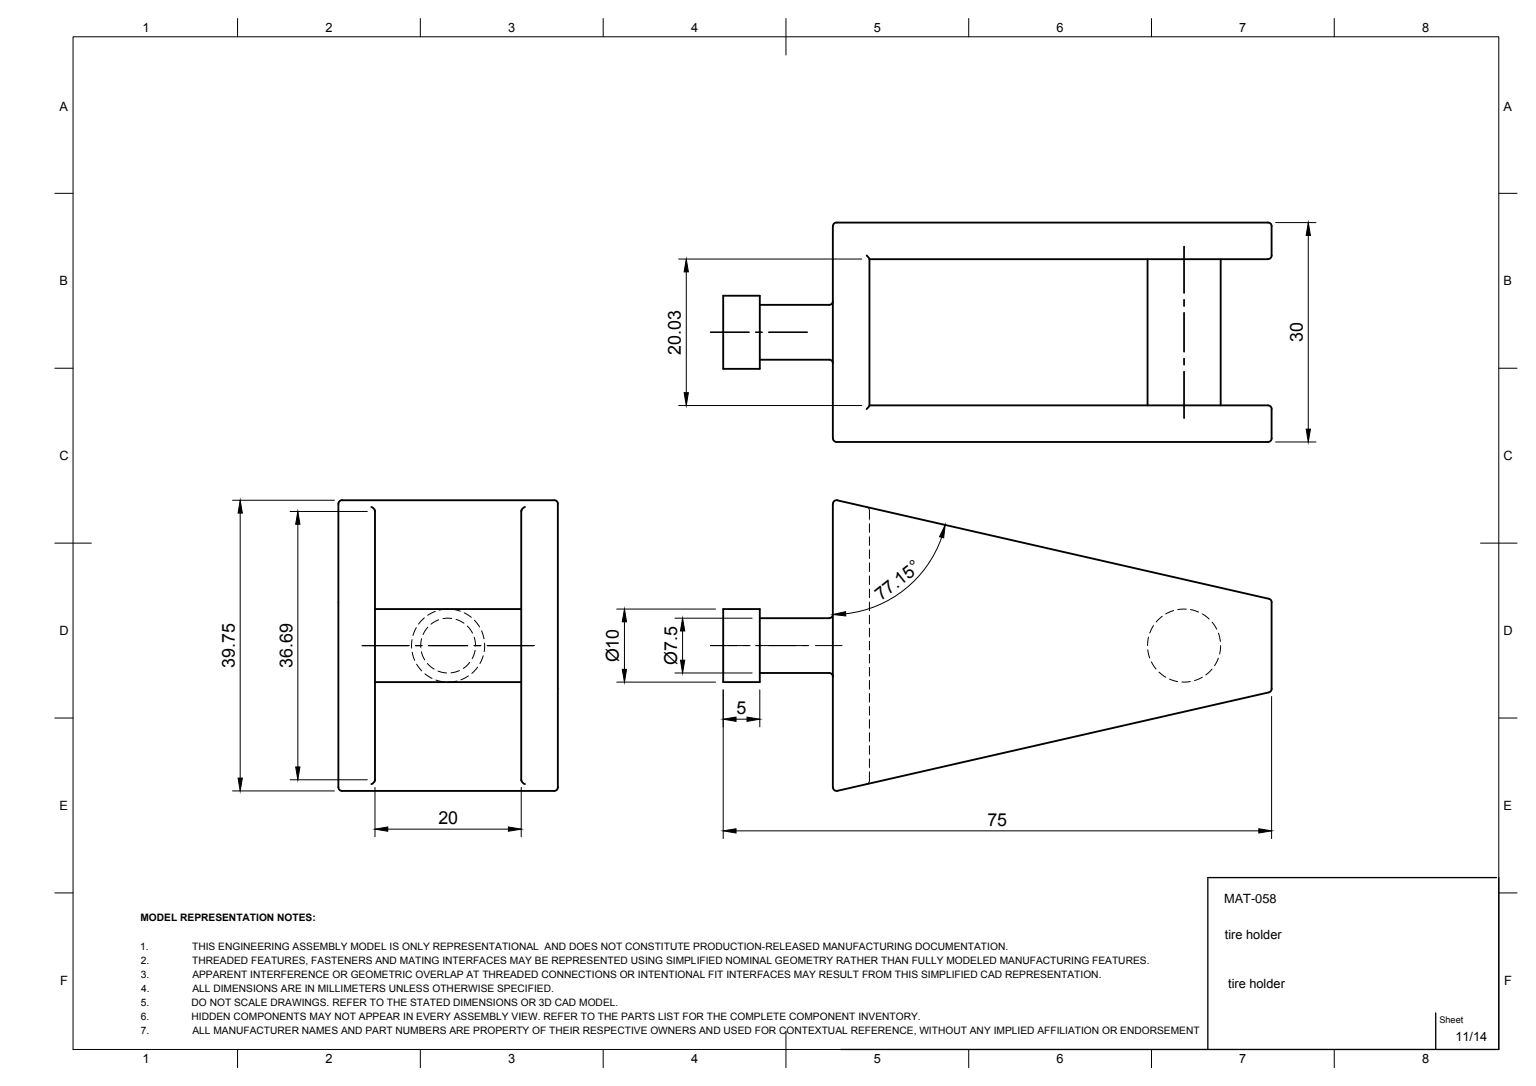
ISO-10303-21;
HEADER;
FILE_DESCRIPTION (('STEP AP214'),
    '1' );
FILE_NAME ('tire holder.step',
    '2026-10-21T17:54:40',
    ( '' ),
    ( '' ),
    'SwSTEP 2.0',
    'SolidWorks 2026',
    '' );
FILE_SCHEMA (( 'AUTOMOTIVE_DESIGN' ));
ENDSEC;

DATA;
#45=LINE ( 'NONE', #24156, #46879 ) ;
#75=DIRECTION ( 'NONE',  ( 0.000000000000000000, 3.469446951953611033E-15, 1.000000000000000000 ) ) ;
#80=CARTESIAN_POINT ( 'NONE',  ( -10.00000000000000355, -34.54492135858216528, 5.000000000000000000 ) ) ;
#120=EDGE_LOOP ( 'NONE', ( #42684, #24578, #28599, #31905 ) ) ;
#171=EDGE_LOOP ( 'NONE', ( #28708, #6316, #9774, #15681 ) ) ;
#207=DIRECTION ( 'NONE',  ( -3.469446951953610639E-15, 0.000000000000000000, 1.000000000000000000 ) ) ;
#240=AXIS2_PLACEMENT_3D ( 'NONE', #22049, #38489, #34625 ) ;
#261=LINE ( 'NONE', #24365, #22339 ) ;
#263=FACE_OUTER_BOUND ( 'NONE', #4989, .T. ) ;
#284=AXIS2_PLACEMENT_3D ( 'NONE', #31805, #27184, #19732 ) ;
#316=AXIS2_PLACEMENT_3D ( 'NONE', #35851, #27117, #42740 ) ;
#348=DIRECTION ( 'NONE',  ( -1.000000000000000000, -0.000000000000000000, -0.000000000000000000 ) ) ;
#396=AXIS2_PLACEMENT_3D ( 'NONE', #30919, #46501, #11395 ) ;
#430=LINE ( 'NONE', #46568, #36748 ) ;
#460=ORIENTED_EDGE ( 'NONE', *, *, #7056, .F. ) ;
#535=FACE_OUTER_BOUND ( 'NONE', #48692, .T. ) ;
#576=VERTEX_POINT ( 'NONE', #29130 ) ;
#579=DIRECTION ( 'NONE',  ( -1.000000000000000000, 0.000000000000000000, 0.000000000000000000 ) ) ;
#589=CARTESIAN_POINT ( 'NONE',  ( -10.49999999999999467, -46.01315789473684248, -5.916985404131818171 ) ) ;
#592=EDGE_CURVE ( 'NONE', #28510, #10704, #32994, .T. ) ;
#599=DIRECTION ( 'NONE',  ( 0.000000000000000000, 0.2223603367690637489, -0.9749645535258953943 ) ) ;
#609=VERTEX_POINT ( 'NONE', #32230 ) ;
#633=FACE_OUTER_BOUND ( 'NONE', #3064, .T. ) ;
#751=FACE_OUTER_BOUND ( 'NONE', #17565, .T. ) ;
#819=EDGE_LOOP ( 'NONE', ( #45356, #48998, #15248, #7254 ) ) ;
#834=LINE ( 'NONE', #43911, #33679 ) ;
#877=CARTESIAN_POINT ( 'NONE',  ( 9.999999999999998224, -41.51315789473684248, -25.00000000000000000 ) ) ;
#894=LINE ( 'NONE', #40643, #19792 ) ;
#895=ORIENTED_EDGE ( 'NONE', *, *, #4687, .F. ) ;
#954=CARTESIAN_POINT ( 'NONE',  ( 10.00419011302946259, 8.486842105263161073, 18.42339408367722697 ) ) ;
#973=CARTESIAN_POINT ( 'NONE',  ( -10.01251772323708522, 8.486842105263161073, -18.46084505325461578 ) ) ;
#990=CARTESIAN_POINT ( 'NONE',  ( 15.00000000000000000, 8.986842105263161073, 18.46084505325461578 ) ) ;
#1024=DIRECTION ( 'NONE',  ( 0.000000000000000000, 0.000000000000000000, -1.000000000000000000 ) ) ;
#1096=DIRECTION ( 'NONE',  ( 1.000000000000000000, -0.000000000000000000, -0.000000000000000000 ) ) ;
#1116=EDGE_CURVE ( 'NONE', #10525, #16010, #26971, .T. ) ;
#1161=VERTEX_POINT ( 'NONE', #21613 ) ;
#1182=SPHERICAL_SURFACE ( 'NONE', #12671, 0.5000000000000000000 ) ;
#1197=DIRECTION ( 'NONE',  ( 0.000000000000000000, -0.000000000000000000, 1.000000000000000000 ) ) ;
#1232=CARTESIAN_POINT ( 'NONE',  ( 14.49999999999999822, 12.98684210526315930, 19.37312575500899925 ) ) ;
#1234=DIRECTION ( 'NONE',  ( -0.000000000000000000, -1.000000000000000000, -0.000000000000000000 ) ) ;
#1240=EDGE_CURVE ( 'NONE', #38020, #13837, #23637, .T. ) ;
#1272=ORIENTED_EDGE ( 'NONE', *, *, #4241, .T. ) ;
#1288=ORIENTED_EDGE ( 'NONE', *, *, #47195, .F. ) ;
#1496=DIRECTION ( 'NONE',  ( 0.000000000000000000, 0.000000000000000000, -1.000000000000000000 ) ) ;
#1555=ORIENTED_EDGE ( 'NONE', *, *, #40015, .F. ) ;
#1561=ADVANCED_FACE ( 'NONE', ( #6652 ), #17704, .T. ) ;
#1634=VECTOR ( 'NONE', #50677, 1000.000000000000000 ) ;
#1646=CIRCLE ( 'NONE', #12289, 0.4999999999999997224 ) ;
#1662=VERTEX_POINT ( 'NONE', #15882 ) ;
#1709=DIRECTION ( 'NONE',  ( 0.000000000000000000, 6.938893903907221278E-15, -1.000000000000000000 ) ) ;
#1723=DIRECTION ( 'NONE',  ( -1.542934785277626909E-15, 0.9749645535258950613, 0.2223603367690656918 ) ) ;
#1780=AXIS2_PLACEMENT_3D ( 'NONE', #25486, #49289, #14172 ) ;
#1792=EDGE_CURVE ( 'NONE', #35881, #24944, #10954, .T. ) ;
#1843=CIRCLE ( 'NONE', #32181, 0.4999999999999997224 ) ;
#1845=ORIENTED_EDGE ( 'NONE', *, *, #9182, .T. ) ;
#1941=DIRECTION ( 'NONE',  ( 0.000000000000000000, 0.000000000000000000, -1.000000000000000000 ) ) ;
#2025=CARTESIAN_POINT ( 'NONE',  ( 4.592425496802573972E-16, 23.48684210526316107, 3.750000000000000000 ) ) ;
#2046=EDGE_LOOP ( 'NONE', ( #43481, #9210, #37838, #21818, #19453, #27829, #8404, #30225 ) ) ;
#2075=ADVANCED_FACE ( 'NONE', ( #43515 ), #35854, .T. ) ;
#2076=ORIENTED_EDGE ( 'NONE', *, *, #10770, .F. ) ;
#2264=CARTESIAN_POINT ( 'NONE',  ( -10.01251772323708700, 8.486842105263161073, 18.46084505325461578 ) ) ;
#2383=CYLINDRICAL_SURFACE ( 'NONE', #27076, 0.5000000000000004441 ) ;
#2455=AXIS2_PLACEMENT_3D ( 'NONE', #15350, #35622, #7647 ) ;
#2478=ORIENTED_EDGE ( 'NONE', *, *, #4027, .F. ) ;
#2494=( BOUNDED_CURVE ( )  B_SPLINE_CURVE ( 3, ( #33761, #6547, #22202, #15008 ),
 .UNSPECIFIED., .F., .F. ) 
 B_SPLINE_CURVE_WITH_KNOTS ( ( 4, 4 ),
 ( 1.346561575685802925, 1.570796326794893671 ),
 .UNSPECIFIED. ) 
 CURVE ( )  GEOMETRIC_REPRESENTATION_ITEM ( )  RATIONAL_B_SPLINE_CURVE ( ( 1.000000000000000000, 0.9958142854328209115, 0.9958142854328209115, 1.000000000000000000 ) ) 
 REPRESENTATION_ITEM ( '' )  );
#2510=ORIENTED_EDGE ( 'NONE', *, *, #26162, .F. ) ;
#2540=AXIS2_PLACEMENT_3D ( 'NONE', #23259, #35857, #19920 ) ;
#2581=DIRECTION ( 'NONE',  ( 1.000000000000000000, -0.000000000000000000, -0.000000000000000000 ) ) ;
#2605=ADVANCED_FACE ( 'NONE', ( #535 ), #28227, .T. ) ;
#2654=VECTOR ( 'NONE', #49924, 1000.000000000000000 ) ;
#2662=ORIENTED_EDGE ( 'NONE', *, *, #17111, .T. ) ;
#2697=CARTESIAN_POINT ( 'NONE',  ( -9.999999999999994671, -46.01315789473684248, -5.916985404131814619 ) ) ;
#2752=DIRECTION ( 'NONE',  ( 0.000000000000000000, 0.000000000000000000, 1.000000000000000000 ) ) ;
#2761=EDGE_CURVE ( 'NONE', #42454, #20304, #29988, .T. ) ;
#2842=CARTESIAN_POINT ( 'NONE',  ( -15.00000000000000000, 12.98684210526315930, -20.00000000000000000 ) ) ;
#2857=LINE ( 'NONE', #42115, #24978 ) ;
#2930=AXIS2_PLACEMENT_3D ( 'NONE', #5505, #48309, #9612 ) ;
#2932=FACE_OUTER_BOUND ( 'NONE', #31942, .T. ) ;
#2933=( BOUNDED_CURVE ( )  B_SPLINE_CURVE ( 3, ( #26666, #25209, #13891, #30775 ),
 .UNSPECIFIED., .F., .F. ) 
 B_SPLINE_CURVE_WITH_KNOTS ( ( 4, 4 ),
 ( 1.570796326794886788, 1.795031077903984418 ),
 .UNSPECIFIED. ) 
 CURVE ( )  GEOMETRIC_REPRESENTATION_ITEM ( )  RATIONAL_B_SPLINE_CURVE ( ( 1.000000000000000000, 0.9958142854328206894, 0.9958142854328206894, 1.000000000000000000 ) ) 
 REPRESENTATION_ITEM ( '' )  );
#2949=SPHERICAL_SURFACE ( 'NONE', #43069, 0.5000000000000000000 ) ;
#2968=EDGE_LOOP ( 'NONE', ( #14933, #7197, #19117, #5943 ) ) ;
#3064=EDGE_LOOP ( 'NONE', ( #38905, #19899, #45220, #15309 ) ) ;
#3066=VERTEX_POINT ( 'NONE', #25504 ) ;
#3104=ORIENTED_EDGE ( 'NONE', *, *, #47830, .T. ) ;
#3173=CYLINDRICAL_SURFACE ( 'NONE', #24749, 0.5000000000000007772 ) ;
#3180=CARTESIAN_POINT ( 'NONE',  ( -14.49999999999999822, 12.98684210526315930, -19.37312575500900280 ) ) ;
#3200=CARTESIAN_POINT ( 'NONE',  ( -10.01251772323708700, 8.486842105263161073, 18.46084505325461578 ) ) ;
#3209=DIRECTION ( 'NONE',  ( 0.000000000000000000, 0.000000000000000000, -1.000000000000000000 ) ) ;
#3241=EDGE_CURVE ( 'NONE', #43437, #39173, #48510, .T. ) ;
#3301=CIRCLE ( 'NONE', #17237, 5.000000000000000000 ) ;
#3396=EDGE_CURVE ( 'NONE', #19221, #42182, #41183, .T. ) ;
#3427=( NAMED_UNIT ( * ) PLANE_ANGLE_UNIT ( ) SI_UNIT ( $, .RADIAN. ) );
#3464=CIRCLE ( 'NONE', #8400, 0.4999999999999995559 ) ;
#3536=EDGE_CURVE ( 'NONE', #24944, #35881, #21519, .T. ) ;
#3663=ORIENTED_EDGE ( 'NONE', *, *, #7740, .F. ) ;
#3712=ORIENTED_EDGE ( 'NONE', *, *, #33824, .F. ) ;
#3728=DIRECTION ( 'NONE',  ( 0.000000000000000000, 0.000000000000000000, 1.000000000000000000 ) ) ;
#3770=CARTESIAN_POINT ( 'NONE',  ( -14.49999999999999822, 13.59802227364769323, -19.51251772323705325 ) ) ;
#3785=ORIENTED_EDGE ( 'NONE', *, *, #26162, .T. ) ;
#3786=EDGE_LOOP ( 'NONE', ( #5766, #9145, #25506, #27864 ) ) ;
#3830=CARTESIAN_POINT ( 'NONE',  ( 10.00000000000000355, -48.43825625180578953, 5.363892796379245986 ) ) ;
#3840=DIRECTION ( 'NONE',  ( -1.000000000000000000, -0.000000000000000000, -0.000000000000000000 ) ) ;
#3855=EDGE_CURVE ( 'NONE', #35640, #27759, #5651, .T. ) ;
#3910=UNCERTAINTY_MEASURE_WITH_UNIT (LENGTH_MEASURE( 1.000000000000000082E-05 ), #38612, 'distance_accuracy_value', 'NONE');
#3932=ORIENTED_EDGE ( 'NONE', *, *, #33759, .F. ) ;
#3990=CARTESIAN_POINT ( 'NONE',  ( 15.00000000000000000, -46.01315789473684248, 0.000000000000000000 ) ) ;
#4021=VECTOR ( 'NONE', #29786, 1000.000000000000000 ) ;
#4027=EDGE_CURVE ( 'NONE', #23110, #34075, #10732, .T. ) ;
#4062=ORIENTED_EDGE ( 'NONE', *, *, #44355, .T. ) ;
#4075=FACE_OUTER_BOUND ( 'NONE', #46172, .T. ) ;
#4085=DIRECTION ( 'NONE',  ( -0.000000000000000000, 1.000000000000000000, 0.000000000000000000 ) ) ;
#4104=FACE_OUTER_BOUND ( 'NONE', #4399, .T. ) ;
#4145=FACE_OUTER_BOUND ( 'NONE', #18052, .T. ) ;
#4234=CYLINDRICAL_SURFACE ( 'NONE', #14707, 0.5000000000000004441 ) ;
#4241=EDGE_CURVE ( 'NONE', #24669, #43437, #22901, .T. ) ;
#4256=ORIENTED_EDGE ( 'NONE', *, *, #50333, .T. ) ;
#4260=AXIS2_PLACEMENT_3D ( 'NONE', #32923, #33666, #24959 ) ;
#4282=CARTESIAN_POINT ( 'NONE',  ( 10.25676241992214877, 8.638513918217338272, 18.89424093979656405 ) ) ;
#4395=DIRECTION ( 'NONE',  ( 0.000000000000000000, -0.2223603367690619725, -0.9749645535258958384 ) ) ;
#4399=EDGE_LOOP ( 'NONE', ( #26499, #28171, #23925, #10924 ) ) ;
#4431=CARTESIAN_POINT ( 'NONE',  ( 15.00000000000000000, 13.48684210526315930, 19.37312575500900280 ) ) ;
#4458=CIRCLE ( 'NONE', #13457, 0.5000000000000004441 ) ;
#4485=VECTOR ( 'NONE', #38359, 1000.000000000000000 ) ;
#4487=ORIENTED_EDGE ( 'NONE', *, *, #20206, .F. ) ;
#4544=LINE ( 'NONE', #24549, #10987 ) ;
#4626=AXIS2_PLACEMENT_3D ( 'NONE', #26012, #29596, #18790 ) ;
#4650=DIRECTION ( 'NONE',  ( 0.000000000000000000, 0.000000000000000000, 1.000000000000000000 ) ) ;
#4687=EDGE_CURVE ( 'NONE', #35926, #43437, #34948, .T. ) ;
#4718=DIRECTION ( 'NONE',  ( 1.000000000000000000, 6.938893903907233308E-16, 0.000000000000000000 ) ) ;
#4758=ORIENTED_EDGE ( 'NONE', *, *, #4027, .T. ) ;
#4779=CARTESIAN_POINT ( 'NONE',  ( 9.999999999999962697, 8.486842105263161073, 18.38522261288946780 ) ) ;
#4828=AXIS2_PLACEMENT_3D ( 'NONE', #3770, #19420, #15572 ) ;
#4835=VECTOR ( 'NONE', #39057, 1000.000000000000000 ) ;
#4900=DIRECTION ( 'NONE',  ( -6.938893903907221278E-15, -0.000000000000000000, -1.000000000000000000 ) ) ;
#4964=DIRECTION ( 'NONE',  ( 0.000000000000000000, -1.000000000000000000, 0.000000000000000000 ) ) ;
#4989=EDGE_LOOP ( 'NONE', ( #24819, #3104, #38758 ) ) ;
#4996=ORIENTED_EDGE ( 'NONE', *, *, #34082, .F. ) ;
#5053=LINE ( 'NONE', #17118, #10391 ) ;
#5074=DIRECTION ( 'NONE',  ( 1.000000000000000000, 0.000000000000000000, -0.000000000000000000 ) ) ;
#5167=AXIS2_PLACEMENT_3D ( 'NONE', #17587, #21943, #1941 ) ;
#5214=( LENGTH_UNIT ( ) NAMED_UNIT ( * ) SI_UNIT ( .MILLI., .METRE. ) );
#5228=DIRECTION ( 'NONE',  ( 0.000000000000000000, -0.9749645535258959494, -0.2223603367690620558 ) ) ;
#5249=ORIENTED_EDGE ( 'NONE', *, *, #39960, .F. ) ;
#5287=AXIS2_PLACEMENT_3D ( 'NONE', #877, #4718, #17016 ) ;
#5349=DIRECTION ( 'NONE',  ( -0.000000000000000000, 1.000000000000000000, 0.000000000000000000 ) ) ;
#5426=VERTEX_POINT ( 'NONE', #29943 ) ;
#5505=CARTESIAN_POINT ( 'NONE',  ( -14.49999999999999822, 12.98684210526315930, 19.37312575500900280 ) ) ;
#5556=VERTEX_POINT ( 'NONE', #32723 ) ;
#5562=DIRECTION ( 'NONE',  ( 0.000000000000000000, -0.2223603367690656640, 0.9749645535258950613 ) ) ;
#5568=EDGE_LOOP ( 'NONE', ( #49170, #12060, #17176 ) ) ;
#5569=DIRECTION ( 'NONE',  ( 0.000000000000000000, 1.000000000000000000, 0.000000000000000000 ) ) ;
#5605=DIRECTION ( 'NONE',  ( -0.000000000000000000, -1.000000000000000000, -0.000000000000000000 ) ) ;
#5606=EDGE_CURVE ( 'NONE', #32346, #49488, #6014, .T. ) ;
#5651=CIRCLE ( 'NONE', #37653, 0.4999999999999997224 ) ;
#5654=DIRECTION ( 'NONE',  ( -1.000000000000000000, 0.000000000000000000, 0.000000000000000000 ) ) ;
#5662=CARTESIAN_POINT ( 'NONE',  ( -14.49999999999999822, -46.01315789473684248, -5.916985404131818171 ) ) ;
#5718=AXIS2_PLACEMENT_3D ( 'NONE', #46898, #5349, #28463 ) ;
#5766=ORIENTED_EDGE ( 'NONE', *, *, #17761, .T. ) ;
#5824=VERTEX_POINT ( 'NONE', #13102 ) ;
#5861=ORIENTED_EDGE ( 'NONE', *, *, #25959, .F. ) ;
#5908=DIRECTION ( 'NONE',  ( -0.000000000000000000, 0.9749645535258953943, 0.2223603367690637489 ) ) ;
#5936=CARTESIAN_POINT ( 'NONE',  ( 10.50000000000000178, -46.12433806312137108, 6.404467680894761372 ) ) ;
#5940=CARTESIAN_POINT ( 'NONE',  ( 10.25676241992214344, 8.638513918217336496, -18.89424093979656760 ) ) ;
#5943=ORIENTED_EDGE ( 'NONE', *, *, #592, .F. ) ;
#6014=LINE ( 'NONE', #24519, #32174 ) ;
#6166=DIRECTION ( 'NONE',  ( -1.000000000000000000, 0.000000000000000000, -0.000000000000000000 ) ) ;
#6187=ORIENTED_EDGE ( 'NONE', *, *, #28725, .T. ) ;
#6196=PRODUCT_DEFINITION_FORMATION_WITH_SPECIFIED_SOURCE ( 'ANY', '', #26565, .NOT_KNOWN. ) ;
#6204=DIRECTION ( 'NONE',  ( 0.000000000000000000, 0.000000000000000000, 1.000000000000000000 ) ) ;
#6271=CARTESIAN_POINT ( 'NONE',  ( 15.00000000000000000, -46.01315789473684248, 5.916985404131816395 ) ) ;
#6278=CIRCLE ( 'NONE', #19373, 0.4999999999999995559 ) ;
#6285=CARTESIAN_POINT ( 'NONE',  ( -10.06660411345808193, 8.486842105263161073, -18.70408263333243326 ) ) ;
#6306=DIRECTION ( 'NONE',  ( -0.000000000000000000, 1.000000000000000000, 0.000000000000000000 ) ) ;
#6316=ORIENTED_EDGE ( 'NONE', *, *, #12510, .F. ) ;
#6317=FACE_OUTER_BOUND ( 'NONE', #44802, .T. ) ;
#6351=ORIENTED_EDGE ( 'NONE', *, *, #3536, .T. ) ;
#6366=CARTESIAN_POINT ( 'NONE',  ( -10.00000000000003375, 8.486842105263161073, 18.38522261288946780 ) ) ;
#6426=ADVANCED_FACE ( 'NONE', ( #7629 ), #43272, .T. ) ;
#6443=VERTEX_POINT ( 'NONE', #46577 ) ;
#6516=CARTESIAN_POINT ( 'NONE',  ( -14.49999999999999822, 12.87566193687862715, -19.86060803177194956 ) ) ;
#6530=AXIS2_PLACEMENT_3D ( 'NONE', #50614, #15762, #11667 ) ;
#6547=CARTESIAN_POINT ( 'NONE',  ( 10.00419011302945904, 8.486842105263161073, -18.42339408367723053 ) ) ;
#6652=FACE_OUTER_BOUND ( 'NONE', #35530, .T. ) ;
#6701=DIRECTION ( 'NONE',  ( 0.000000000000000000, 0.000000000000000000, -1.000000000000000000 ) ) ;
#6724=EDGE_LOOP ( 'NONE', ( #17001, #30815, #36441 ) ) ;
#6731=ORIENTED_EDGE ( 'NONE', *, *, #11598, .F. ) ;
#6774=CARTESIAN_POINT ( 'NONE',  ( 10.50000000000000178, -46.01315789473684248, -5.916985404131818171 ) ) ;
#6799=CARTESIAN_POINT ( 'NONE',  ( 0.000000000000000000, 23.48684210526316107, 0.000000000000000000 ) ) ;
#6871=DIRECTION ( 'NONE',  ( 0.000000000000000000, -1.000000000000000000, 0.000000000000000000 ) ) ;
#6885=CARTESIAN_POINT ( 'NONE',  ( 9.999999999999998224, 8.486842105263161073, 18.46084505325461933 ) ) ;
#6895=CARTESIAN_POINT ( 'NONE',  ( 9.999999999999998224, 8.486842105263161073, -18.46084505325461578 ) ) ;
#6946=DIRECTION ( 'NONE',  ( 6.938893903907233308E-16, -1.000000000000000000, 0.000000000000000000 ) ) ;
#6954=AXIS2_PLACEMENT_3D ( 'NONE', #9415, #12996, #49122 ) ;
#6956=ORIENTED_EDGE ( 'NONE', *, *, #7114, .F. ) ;
#6977=AXIS2_PLACEMENT_3D ( 'NONE', #21956, #45271, #37879 ) ;
#6998=AXIS2_PLACEMENT_3D ( 'NONE', #21667, #49075, #29623 ) ;
#7040=VECTOR ( 'NONE', #15019, 1000.000000000000000 ) ;
#7052=CARTESIAN_POINT ( 'NONE',  ( 4.592425496802573972E-16, 13.98684210526316107, 3.750000000000000000 ) ) ;
#7056=EDGE_CURVE ( 'NONE', #38020, #1662, #894, .T. ) ;
#7062=EDGE_CURVE ( 'NONE', #35881, #31952, #32188, .T. ) ;
#7084=ORIENTED_EDGE ( 'NONE', *, *, #10641, .F. ) ;
#7113=EDGE_CURVE ( 'NONE', #7866, #1662, #37840, .T. ) ;
#7114=EDGE_CURVE ( 'NONE', #20701, #39523, #30456, .T. ) ;
#7197=ORIENTED_EDGE ( 'NONE', *, *, #25233, .F. ) ;
#7202=DIRECTION ( 'NONE',  ( -1.000000000000000000, -6.938893903907233308E-16, 0.000000000000000000 ) ) ;
#7254=ORIENTED_EDGE ( 'NONE', *, *, #24579, .F. ) ;
#7273=EDGE_CURVE ( 'NONE', #28229, #5824, #15967, .T. ) ;
#7275=FACE_OUTER_BOUND ( 'NONE', #21467, .T. ) ;
#7324=ORIENTED_EDGE ( 'NONE', *, *, #31534, .F. ) ;
#7325=EDGE_LOOP ( 'NONE', ( #22359, #3712, #17058, #14186 ) ) ;
#7392=EDGE_LOOP ( 'NONE', ( #23020, #17478, #31410, #21280 ) ) ;
#7412=ORIENTED_EDGE ( 'NONE', *, *, #24326, .T. ) ;
#7417=EDGE_CURVE ( 'NONE', #16010, #39173, #12121, .T. ) ;
#7478=EDGE_CURVE ( 'NONE', #39523, #20701, #16513, .T. ) ;
#7479=CARTESIAN_POINT ( 'NONE',  ( 15.00000000000000000, -46.12433806312137108, -6.404467680894764925 ) ) ;
#7526=CARTESIAN_POINT ( 'NONE',  ( 15.00000000000000000, -3.557843729863134463, -15.59977635401528850 ) ) ;
#7618=AXIS2_PLACEMENT_3D ( 'NONE', #12378, #348, #43665 ) ;
#7629=FACE_OUTER_BOUND ( 'NONE', #7392, .T. ) ;
#7647=DIRECTION ( 'NONE',  ( 0.000000000000000000, 0.2223603367690619725, -0.9749645535258958384 ) ) ;
#7664=EDGE_CURVE ( 'NONE', #34755, #31952, #12256, .T. ) ;
#7676=DIRECTION ( 'NONE',  ( 1.000000000000000000, 0.000000000000000000, -1.734723475976805517E-15 ) ) ;
#7703=AXIS2_PLACEMENT_3D ( 'NONE', #8195, #4085, #8448 ) ;
#7731=ORIENTED_EDGE ( 'NONE', *, *, #23304, .T. ) ;
#7733=DIRECTION ( 'NONE',  ( -0.000000000000000000, 0.000000000000000000, -1.000000000000000000 ) ) ;
#7740=EDGE_CURVE ( 'NONE', #13837, #42454, #28716, .T. ) ;
#7746=DIRECTION ( 'NONE',  ( 1.542934785277601468E-15, 0.9749645535258959494, -0.2223603367690620558 ) ) ;
#7780=CIRCLE ( 'NONE', #36463, 0.5000000000000000000 ) ;
#7798=DIRECTION ( 'NONE',  ( 6.765175596986472868E-16, -0.9749645535258953943, -0.2223603367690637489 ) ) ;
#7806=LINE ( 'NONE', #43436, #23351 ) ;
#7809=ORIENTED_EDGE ( 'NONE', *, *, #25233, .T. ) ;
#7813=DIRECTION ( 'NONE',  ( 0.000000000000000000, 0.000000000000000000, 1.000000000000000000 ) ) ;
#7820=CARTESIAN_POINT ( 'NONE',  ( -14.49999999999999822, -46.51315789473684248, -5.916985404131818171 ) ) ;
#7828=LINE ( 'NONE', #35042, #44206 ) ;
#7829=ORIENTED_EDGE ( 'NONE', *, *, #36041, .T. ) ;
#7842=ORIENTED_EDGE ( 'NONE', *, *, #44186, .T. ) ;
#7866=VERTEX_POINT ( 'NONE', #30673 ) ;
#7886=AXIS2_PLACEMENT_3D ( 'NONE', #1232, #1723, #5562 ) ;
#7900=FACE_OUTER_BOUND ( 'NONE', #31199, .T. ) ;
#7910=VECTOR ( 'NONE', #1096, 1000.000000000000000 ) ;
#7922=ORIENTED_EDGE ( 'NONE', *, *, #13439, .T. ) ;
#8033=DIRECTION ( 'NONE',  ( 0.000000000000000000, 0.000000000000000000, 1.000000000000000000 ) ) ;
#8051=ADVANCED_FACE ( 'NONE', ( #47541 ), #4234, .T. ) ;
#8052=EDGE_CURVE ( 'NONE', #40121, #28181, #11932, .T. ) ;
#8082=EDGE_LOOP ( 'NONE', ( #35213, #15987, #29822, #26821, #47039, #4758, #23954, #45682 ) ) ;
#8195=CARTESIAN_POINT ( 'NONE',  ( 14.49999999999999822, -46.01315789473684248, 5.916985404131813731 ) ) ;
#8236=VERTEX_POINT ( 'NONE', #33954 ) ;
#8245=DIRECTION ( 'NONE',  ( -1.000000000000000000, 0.000000000000000000, 0.000000000000000000 ) ) ;
#8352=DIRECTION ( 'NONE',  ( 0.000000000000000000, 8.673617379884027583E-15, 1.000000000000000000 ) ) ;
#8358=ORIENTED_EDGE ( 'NONE', *, *, #46516, .F. ) ;
#8400=AXIS2_PLACEMENT_3D ( 'NONE', #50720, #35396, #28186 ) ;
#8402=EDGE_LOOP ( 'NONE', ( #48506, #22576, #41484 ) ) ;
#8404=ORIENTED_EDGE ( 'NONE', *, *, #23196, .T. ) ;
#8407=AXIS2_PLACEMENT_3D ( 'NONE', #16644, #35162, #43084 ) ;
#8416=EDGE_CURVE ( 'NONE', #12918, #28229, #15215, .T. ) ;
#8440=CARTESIAN_POINT ( 'NONE',  ( -10.49999999999999467, -46.01315789473684248, 5.916985404131814619 ) ) ;
#8448=DIRECTION ( 'NONE',  ( 3.469446951953616950E-15, 0.000000000000000000, -1.000000000000000000 ) ) ;
#8470=DIRECTION ( 'NONE',  ( 0.000000000000000000, 0.000000000000000000, 1.000000000000000000 ) ) ;
#8504=EDGE_CURVE ( 'NONE', #12400, #26840, #1646, .T. ) ;
#8514=CIRCLE ( 'NONE', #15903, 0.5000000000000004441 ) ;
#8582=DIRECTION ( 'NONE',  ( 6.765175596986471882E-16, -0.9749645535258953943, -0.2223603367690637489 ) ) ;
#8678=DIRECTION ( 'NONE',  ( 0.000000000000000000, 0.2223603367690656640, 0.9749645535258950613 ) ) ;
#8706=UNCERTAINTY_MEASURE_WITH_UNIT (LENGTH_MEASURE( 1.000000000000000082E-05 ), #5214, 'distance_accuracy_value', 'NONE');
#8869=ORIENTED_EDGE ( 'NONE', *, *, #24926, .F. ) ;
#8880=EDGE_CURVE ( 'NONE', #31952, #34755, #39343, .T. ) ;
#8920=DIRECTION ( 'NONE',  ( 0.000000000000000000, 0.000000000000000000, 1.000000000000000000 ) ) ;
#8941=CARTESIAN_POINT ( 'NONE',  ( 10.50000000000000178, -46.01315789473684248, -5.916985404131818171 ) ) ;
#8967=DIRECTION ( 'NONE',  ( 0.000000000000000000, 1.000000000000000000, -0.000000000000000000 ) ) ;
#8972=ADVANCED_FACE ( 'NONE', ( #18419 ), #25886, .T. ) ;
#9003=AXIS2_PLACEMENT_3D ( 'NONE', #31247, #43526, #30993 ) ;
#9016=ORIENTED_EDGE ( 'NONE', *, *, #11598, .T. ) ;
#9033=DIRECTION ( 'NONE',  ( -1.542934785277601468E-15, -0.9749645535258959494, 0.2223603367690620558 ) ) ;
#9040=CARTESIAN_POINT ( 'NONE',  ( 14.49999999999999822, 12.98684210526315930, -19.87312575500900280 ) ) ;
#9100=EDGE_CURVE ( 'NONE', #576, #5426, #31909, .T. ) ;
#9103=ORIENTED_EDGE ( 'NONE', *, *, #33702, .F. ) ;
#9111=ORIENTED_EDGE ( 'NONE', *, *, #23050, .T. ) ;
#9145=ORIENTED_EDGE ( 'NONE', *, *, #14539, .F. ) ;
#9163=DIRECTION ( 'NONE',  ( 1.000000000000000000, 0.000000000000000000, 0.000000000000000000 ) ) ;
#9182=EDGE_CURVE ( 'NONE', #5824, #26840, #26050, .T. ) ;
#9195=DIRECTION ( 'NONE',  ( -1.224646799147352468E-16, 0.000000000000000000, -1.000000000000000000 ) ) ;
#9210=ORIENTED_EDGE ( 'NONE', *, *, #25817, .T. ) ;
#9211=SPHERICAL_SURFACE ( 'NONE', #29493, 0.5000000000000000000 ) ;
#9268=CIRCLE ( 'NONE', #28932, 0.5000000000000004441 ) ;
#9298=PLANE ( 'NONE',  #30473 ) ;
#9406=ORIENTED_EDGE ( 'NONE', *, *, #29481, .T. ) ;
#9415=CARTESIAN_POINT ( 'NONE',  ( 15.00000000000000000, 12.98684210526315752, 19.37312575500900280 ) ) ;
#9419=DIRECTION ( 'NONE',  ( 0.000000000000000000, 0.000000000000000000, 1.000000000000000000 ) ) ;
#9431=CYLINDRICAL_SURFACE ( 'NONE', #38867, 0.5000000000000004441 ) ;
#9438=STYLED_ITEM('',(#50775),#22320);
#9462=DIRECTION ( 'NONE',  ( -1.000000000000000000, 0.000000000000000000, -0.000000000000000000 ) ) ;
#9479=VERTEX_POINT ( 'NONE', #20570 ) ;
#9512=DIRECTION ( 'NONE',  ( -1.000000000000000000, 0.000000000000000000, 6.938893903907222067E-15 ) ) ;
#9543=CARTESIAN_POINT ( 'NONE',  ( 15.00000000000000000, -46.01315789473684248, -5.916985404131813731 ) ) ;
#9570=EDGE_CURVE ( 'NONE', #19221, #30619, #25947, .T. ) ;
#9612=DIRECTION ( 'NONE',  ( 0.000000000000000000, 0.000000000000000000, 1.000000000000000000 ) ) ;
#9626=DIRECTION ( 'NONE',  ( 0.000000000000000000, 0.000000000000000000, 1.000000000000000000 ) ) ;
#9628=CARTESIAN_POINT ( 'NONE',  ( -15.00000000000000000, 13.59802227364770388, 19.51251772323705325 ) ) ;
#9651=DIRECTION ( 'NONE',  ( 1.000000000000000000, -0.000000000000000000, 0.000000000000000000 ) ) ;
#9717=CYLINDRICAL_SURFACE ( 'NONE', #12761, 5.000000000000000000 ) ;
#9731=PRODUCT_DEFINITION_SHAPE ( 'NONE', 'NONE',  #48451 ) ;
#9760=EDGE_LOOP ( 'NONE', ( #39795, #29788, #24517 ) ) ;
#9774=ORIENTED_EDGE ( 'NONE', *, *, #34082, .T. ) ;
#9854=CIRCLE ( 'NONE', #2455, 0.4999999999999997224 ) ;
#9855=EDGE_CURVE ( 'NONE', #20536, #16093, #25815, .T. ) ;
#9859=CIRCLE ( 'NONE', #38563, 0.4999999999999997224 ) ;
#9882=ADVANCED_FACE ( 'NONE', ( #6317 ), #2949, .T. ) ;
#9892=CIRCLE ( 'NONE', #26276, 0.5000000000000004441 ) ;
#9915=LINE ( 'NONE', #26074, #11981 ) ;
#9920=ORIENTED_EDGE ( 'NONE', *, *, #21525, .T. ) ;
#9935=DIRECTION ( 'NONE',  ( 1.000000000000000000, -0.000000000000000000, 0.000000000000000000 ) ) ;
#10004=DIRECTION ( 'NONE',  ( 0.000000000000000000, 0.000000000000000000, -1.000000000000000000 ) ) ;
#10043=CIRCLE ( 'NONE', #44447, 0.5000000000000004441 ) ;
#10057=DIRECTION ( 'NONE',  ( -0.000000000000000000, 0.2223603367690637489, 0.9749645535258953943 ) ) ;
#10074=ORIENTED_EDGE ( 'NONE', *, *, #26140, .F. ) ;
#10145=AXIS2_PLACEMENT_3D ( 'NONE', #47407, #12298, #20256 ) ;
#10180=EDGE_LOOP ( 'NONE', ( #15997, #36779, #31571 ) ) ;
#10233=CARTESIAN_POINT ( 'NONE',  ( 10.50000000000000178, -46.51315789473684248, -6.315789473684215949 ) ) ;
#10259=ADVANCED_FACE ( 'NONE', ( #18040 ), #49300, .T. ) ;
#10272=CARTESIAN_POINT ( 'NONE',  ( -14.49999999999999822, -46.01315789473684248, 5.916985404131814619 ) ) ;
#10286=MECHANICAL_DESIGN_GEOMETRIC_PRESENTATION_REPRESENTATION('',(#9438),#44644);
#10293=CARTESIAN_POINT ( 'NONE',  ( -9.999999999999998224, -41.51315789473684248, -25.00000000000000000 ) ) ;
#10297=ORIENTED_EDGE ( 'NONE', *, *, #15258, .F. ) ;
#10323=DIRECTION ( 'NONE',  ( -1.000000000000000000, -6.938893903907233308E-16, -0.000000000000000000 ) ) ;
#10327=ORIENTED_EDGE ( 'NONE', *, *, #8416, .T. ) ;
#10353=AXIS2_PLACEMENT_3D ( 'NONE', #30370, #14459, #35245 ) ;
#10386=ORIENTED_EDGE ( 'NONE', *, *, #23322, .F. ) ;
#10391=VECTOR ( 'NONE', #1234, 1000.000000000000000 ) ;
#10399=DIRECTION ( 'NONE',  ( -0.000000000000000000, -0.000000000000000000, -1.000000000000000000 ) ) ;
#10404=ORIENTED_EDGE ( 'NONE', *, *, #36343, .F. ) ;
#10459=ORIENTED_EDGE ( 'NONE', *, *, #1792, .T. ) ;
#10525=VERTEX_POINT ( 'NONE', #9040 ) ;
#10530=CARTESIAN_POINT ( 'NONE',  ( 15.00000000000000000, -46.51315789473684248, 5.916985404131814619 ) ) ;
#10638=VECTOR ( 'NONE', #27007, 1000.000000000000000 ) ;
#10641=EDGE_CURVE ( 'NONE', #28669, #5426, #50460, .T. ) ;
#10704=VERTEX_POINT ( 'NONE', #49499 ) ;
#10732=LINE ( 'NONE', #6895, #36012 ) ;
#10770=EDGE_CURVE ( 'NONE', #37345, #5556, #6278, .T. ) ;
#10775=DIRECTION ( 'NONE',  ( 0.000000000000000000, -0.000000000000000000, -1.000000000000000000 ) ) ;
#10820=DIRECTION ( 'NONE',  ( 1.000000000000000000, -0.000000000000000000, 0.000000000000000000 ) ) ;
#10924=ORIENTED_EDGE ( 'NONE', *, *, #23317, .F. ) ;
#10954=CIRCLE ( 'NONE', #39648, 3.750000000000000000 ) ;
#10987=VECTOR ( 'NONE', #40201, 1000.000000000000000 ) ;
#11142=EDGE_LOOP ( 'NONE', ( #41161, #38667, #41903, #7324, #21124 ) ) ;
#11154=DIRECTION ( 'NONE',  ( 0.000000000000000000, 0.9749645535258955054, -0.2223603367690637767 ) ) ;
#11169=VECTOR ( 'NONE', #18997, 1000.000000000000000 ) ;
#11227=ORIENTED_EDGE ( 'NONE', *, *, #3396, .F. ) ;
#11265=LINE ( 'NONE', #30769, #37062 ) ;
#11293=PLANE ( 'NONE',  #45383 ) ;
#11395=DIRECTION ( 'NONE',  ( 0.000000000000000000, 0.000000000000000000, -1.000000000000000000 ) ) ;
#11437=LINE ( 'NONE', #35072, #24295 ) ;
#11518=VECTOR ( 'NONE', #26750, 1000.000000000000000 ) ;
#11532=ORIENTED_EDGE ( 'NONE', *, *, #3241, .F. ) ;
#11558=CARTESIAN_POINT ( 'NONE',  ( 15.00000000000000000, 12.98684210526315752, 19.37312575500900280 ) ) ;
#11598=EDGE_CURVE ( 'NONE', #34075, #28181, #39966, .T. ) ;
#11613=ORIENTED_EDGE ( 'NONE', *, *, #17860, .F. ) ;
#11655=VERTEX_POINT ( 'NONE', #9543 ) ;
#11667=DIRECTION ( 'NONE',  ( 0.000000000000000000, 0.000000000000000000, -1.000000000000000000 ) ) ;
#11783=CARTESIAN_POINT ( 'NONE',  ( -14.49999999999999822, -46.12433806312137108, -6.404467680894764925 ) ) ;
#11785=DIRECTION ( 'NONE',  ( 0.000000000000000000, -0.9749645535258959494, 0.2223603367690620558 ) ) ;
#11853=CARTESIAN_POINT ( 'NONE',  ( 14.49999999999999822, 12.98684210526315752, 19.87312575500900280 ) ) ;
#11923=FACE_OUTER_BOUND ( 'NONE', #23963, .T. ) ;
#11932=LINE ( 'NONE', #23983, #25371 ) ;
#11981=VECTOR ( 'NONE', #41470, 1000.000000000000000 ) ;
#12002=ORIENTED_EDGE ( 'NONE', *, *, #33824, .T. ) ;
#12044=SPHERICAL_SURFACE ( 'NONE', #16696, 0.5000000000000000000 ) ;
#12060=ORIENTED_EDGE ( 'NONE', *, *, #15503, .T. ) ;
#12093=CARTESIAN_POINT ( 'NONE',  ( 15.00000000000000000, 0.000000000000000000, 0.000000000000000000 ) ) ;
#12121=LINE ( 'NONE', #47474, #32078 ) ;
#12205=EDGE_LOOP ( 'NONE', ( #4062, #30291, #30381 ) ) ;
#12231=DIRECTION ( 'NONE',  ( 0.000000000000000000, -0.000000000000000000, 1.000000000000000000 ) ) ;
#12256=CIRCLE ( 'NONE', #9003, 3.750000000000000000 ) ;
#12289=AXIS2_PLACEMENT_3D ( 'NONE', #589, #9033, #48481 ) ;
#12298=DIRECTION ( 'NONE',  ( 0.000000000000000000, 0.000000000000000000, -1.000000000000000000 ) ) ;
#12378=CARTESIAN_POINT ( 'NONE',  ( -10.49999999999999467, -46.01315789473684248, 5.916985404131813731 ) ) ;
#12397=ORIENTED_EDGE ( 'NONE', *, *, #1240, .F. ) ;
#12400=VERTEX_POINT ( 'NONE', #19188 ) ;
#12407=FACE_BOUND ( 'NONE', #28364, .T. ) ;
#12415=EDGE_LOOP ( 'NONE', ( #11613, #14700, #33107, #9920 ) ) ;
#12510=EDGE_CURVE ( 'NONE', #46117, #30636, #3301, .T. ) ;
#12570=EDGE_LOOP ( 'NONE', ( #40357, #29917, #2076, #5249 ) ) ;
#12592=CARTESIAN_POINT ( 'NONE',  ( 15.00000000000000000, 12.87566193687862715, -19.86060803177194956 ) ) ;
#12641=DIRECTION ( 'NONE',  ( -0.000000000000000000, -0.9749645535258953943, 0.2223603367690637489 ) ) ;
#12671=AXIS2_PLACEMENT_3D ( 'NONE', #16315, #28117, #24279 ) ;
#12691=CARTESIAN_POINT ( 'NONE',  ( -9.999999999999998224, 8.486842105263161073, 18.34680996553531784 ) ) ;
#12738=AXIS2_PLACEMENT_3D ( 'NONE', #41734, #41986, #41483 ) ;
#12761=AXIS2_PLACEMENT_3D ( 'NONE', #30166, #25133, #1024 ) ;
#12814=FACE_OUTER_BOUND ( 'NONE', #40158, .T. ) ;
#12846=CYLINDRICAL_SURFACE ( 'NONE', #18474, 0.5000000000000004441 ) ;
#12865=LINE ( 'NONE', #28772, #38883 ) ;
#12918=VERTEX_POINT ( 'NONE', #14102 ) ;
#12963=ADVANCED_FACE ( 'NONE', ( #48710 ), #29513, .T. ) ;
#12982=CARTESIAN_POINT ( 'NONE',  ( 14.49999999999999822, 12.98684210526315930, -19.37312575500900280 ) ) ;
#12996=DIRECTION ( 'NONE',  ( -1.000000000000000000, 0.000000000000000000, 0.000000000000000000 ) ) ;
#12997=CARTESIAN_POINT ( 'NONE',  ( 10.49999999999996447, 8.875661936878630698, 18.94832733001756253 ) ) ;
#13004=CYLINDRICAL_SURFACE ( 'NONE', #29247, 0.5000000000000004441 ) ;
#13059=DIRECTION ( 'NONE',  ( 0.000000000000000000, 0.000000000000000000, -1.000000000000000000 ) ) ;
#13079=AXIS2_PLACEMENT_3D ( 'NONE', #25938, #26422, #26179 ) ;
#13102=CARTESIAN_POINT ( 'NONE',  ( -9.999999999999994671, -46.01315789473684248, 5.916985404131813731 ) ) ;
#13145=CARTESIAN_POINT ( 'NONE',  ( 15.00000000000000000, 13.48684210526315930, -20.00000000000000000 ) ) ;
#13187=ORIENTED_EDGE ( 'NONE', *, *, #33064, .F. ) ;
#13228=SPHERICAL_SURFACE ( 'NONE', #21290, 0.5000000000000000000 ) ;
#13305=FACE_OUTER_BOUND ( 'NONE', #40318, .T. ) ;
#13333=AXIS2_PLACEMENT_3D ( 'NONE', #45347, #29732, #22025 ) ;
#13343=LINE ( 'NONE', #39813, #36532 ) ;
#13430=ADVANCED_FACE ( 'NONE', ( #38940 ), #50670, .T. ) ;
#13439=EDGE_CURVE ( 'NONE', #19764, #42454, #45458, .T. ) ;
#13455=DIRECTION ( 'NONE',  ( 0.000000000000000000, -0.9749645535258953943, -0.2223603367690637489 ) ) ;
#13457=AXIS2_PLACEMENT_3D ( 'NONE', #8440, #47130, #7676 ) ;
#13533=( GEOMETRIC_REPRESENTATION_CONTEXT ( 3 ) GLOBAL_UNCERTAINTY_ASSIGNED_CONTEXT ( ( #3910 ) ) GLOBAL_UNIT_ASSIGNED_CONTEXT ( ( #38612, #3427, #30914 ) ) REPRESENTATION_CONTEXT ( 'NONE', 'WORKASPACE' ) );
#13561=DIRECTION ( 'NONE',  ( -0.000000000000000000, -1.000000000000000000, -0.000000000000000000 ) ) ;
#13577=AXIS2_PLACEMENT_3D ( 'NONE', #19777, #24408, #27488 ) ;
#13593=ORIENTED_EDGE ( 'NONE', *, *, #28633, .F. ) ;
#13606=CARTESIAN_POINT ( 'NONE',  ( 15.00000000000000000, -46.01315789473684248, -5.916985404131818171 ) ) ;
#13649=CIRCLE ( 'NONE', #34074, 0.5000000000000004441 ) ;
#13680=LINE ( 'NONE', #44946, #31163 ) ;
#13702=DIRECTION ( 'NONE',  ( 1.000000000000000000, -0.000000000000000000, -0.000000000000000000 ) ) ;
#13774=FACE_OUTER_BOUND ( 'NONE', #32709, .T. ) ;
#13832=DIRECTION ( 'NONE',  ( -0.000000000000000000, -1.000000000000000000, -0.000000000000000000 ) ) ;
#13837=VERTEX_POINT ( 'NONE', #47969 ) ;
#13871=ORIENTED_EDGE ( 'NONE', *, *, #7664, .T. ) ;
#13884=FACE_OUTER_BOUND ( 'NONE', #19931, .T. ) ;
#13886=EDGE_CURVE ( 'NONE', #42504, #46782, #47436, .T. ) ;
#13891=CARTESIAN_POINT ( 'NONE',  ( -10.00419011302953010, 8.486842105263161073, -18.42339408367722697 ) ) ;
#13943=EDGE_LOOP ( 'NONE', ( #19817, #7842, #32479, #7731 ) ) ;
#13958=CARTESIAN_POINT ( 'NONE',  ( -10.50000000000003375, 8.875661936878628921, -18.94832733001756253 ) ) ;
#13997=EDGE_CURVE ( 'NONE', #35640, #30619, #47478, .T. ) ;
#14027=AXIS2_PLACEMENT_3D ( 'NONE', #32240, #1197, #16078 ) ;
#14102=CARTESIAN_POINT ( 'NONE',  ( -9.999999999999998224, 8.486842105263161073, -18.34680996553531784 ) ) ;
#14129=ORIENTED_EDGE ( 'NONE', *, *, #8052, .F. ) ;
#14135=DIRECTION ( 'NONE',  ( 1.000000000000000000, -0.000000000000000000, -0.000000000000000000 ) ) ;
#14172=DIRECTION ( 'NONE',  ( -1.000000000000000000, 0.000000000000000000, 0.000000000000000000 ) ) ;
#14185=ADVANCED_FACE ( 'NONE', ( #263 ), #15641, .T. ) ;
#14186=ORIENTED_EDGE ( 'NONE', *, *, #23501, .F. ) ;
#14229=CARTESIAN_POINT ( 'NONE',  ( -9.999999999999994671, -46.01315789473684248, -25.00000000000000000 ) ) ;
#14378=DIRECTION ( 'NONE',  ( 0.000000000000000000, -1.000000000000000000, 0.000000000000000000 ) ) ;
#14428=CARTESIAN_POINT ( 'NONE',  ( 14.49999999999999822, -46.12433806312137108, 6.404467680894761372 ) ) ;
#14459=DIRECTION ( 'NONE',  ( -1.000000000000000000, 0.000000000000000000, 0.000000000000000000 ) ) ;
#14539=EDGE_CURVE ( 'NONE', #43275, #37697, #34846, .T. ) ;
#14570=EDGE_LOOP ( 'NONE', ( #46340, #8869, #18825, #38854 ) ) ;
#14599=ADVANCED_FACE ( 'NONE', ( #23788 ), #40194, .T. ) ;
#14685=FACE_OUTER_BOUND ( 'NONE', #49360, .T. ) ;
#14700=ORIENTED_EDGE ( 'NONE', *, *, #23322, .T. ) ;
#14707=AXIS2_PLACEMENT_3D ( 'NONE', #15519, #26818, #22953 ) ;
#14711=FACE_OUTER_BOUND ( 'NONE', #12570, .T. ) ;
#14739=ORIENTED_EDGE ( 'NONE', *, *, #32162, .T. ) ;
#14750=FACE_BOUND ( 'NONE', #28963, .T. ) ;
#14785=ORIENTED_EDGE ( 'NONE', *, *, #7273, .T. ) ;
#14836=DIRECTION ( 'NONE',  ( 0.000000000000000000, 0.000000000000000000, 1.000000000000000000 ) ) ;
#14933=ORIENTED_EDGE ( 'NONE', *, *, #36920, .T. ) ;
#15008=CARTESIAN_POINT ( 'NONE',  ( 9.999999999999998224, 8.486842105263161073, -18.34680996553532140 ) ) ;
#15019=DIRECTION ( 'NONE',  ( 1.000000000000000000, -0.000000000000000000, -0.000000000000000000 ) ) ;
#15056=DIRECTION ( 'NONE',  ( 6.765175596986471882E-16, -0.9749645535258953943, 0.2223603367690637489 ) ) ;
#15215=LINE ( 'NONE', #34468, #10638 ) ;
#15248=ORIENTED_EDGE ( 'NONE', *, *, #13997, .F. ) ;
#15258=EDGE_CURVE ( 'NONE', #24669, #39173, #35305, .T. ) ;
#15297=EDGE_CURVE ( 'NONE', #30636, #20701, #834, .T. ) ;
#15301=CARTESIAN_POINT ( 'NONE',  ( -10.00000000000000355, -34.54492135858216528, 0.000000000000000000 ) ) ;
#15309=ORIENTED_EDGE ( 'NONE', *, *, #29481, .F. ) ;
#15319=CARTESIAN_POINT ( 'NONE',  ( 14.49999999999999822, -46.51315789473684248, -6.315789473684215949 ) ) ;
#15350=CARTESIAN_POINT ( 'NONE',  ( 14.49999999999999822, -46.01315789473684248, 5.916985404131816395 ) ) ;
#15356=DIRECTION ( 'NONE',  ( 0.000000000000000000, 1.000000000000000000, 0.000000000000000000 ) ) ;
#15371=SPHERICAL_SURFACE ( 'NONE', #18599, 0.5000000000000000000 ) ;
#15418=EDGE_CURVE ( 'NONE', #20304, #28229, #50079, .T. ) ;
#15435=CIRCLE ( 'NONE', #23640, 0.5000000000000004441 ) ;
#15503=EDGE_CURVE ( 'NONE', #5556, #28357, #9892, .T. ) ;
#15519=CARTESIAN_POINT ( 'NONE',  ( 15.00000000000000000, -46.01315789473684248, 5.916985404131814619 ) ) ;
#15572=DIRECTION ( 'NONE',  ( 0.000000000000000000, -0.2223603367690656640, -0.9749645535258950613 ) ) ;
#15616=CARTESIAN_POINT ( 'NONE',  ( -14.49999999999999822, -46.01315789473684248, 5.916985404131813731 ) ) ;
#15641=SPHERICAL_SURFACE ( 'NONE', #5718, 0.5000000000000000000 ) ;
#15647=CARTESIAN_POINT ( 'NONE',  ( 0.000000000000000000, 23.48684210526316107, -5.000000000000000000 ) ) ;
#15652=CYLINDRICAL_SURFACE ( 'NONE', #17189, 0.5000000000000004441 ) ;
#15654=ORIENTED_EDGE ( 'NONE', *, *, #38408, .F. ) ;
#15681=ORIENTED_EDGE ( 'NONE', *, *, #7478, .T. ) ;
#15699=CARTESIAN_POINT ( 'NONE',  ( -14.49999999999999822, 13.48684210526315930, -20.00000000000000000 ) ) ;
#15762=DIRECTION ( 'NONE',  ( -0.000000000000000000, -1.000000000000000000, -0.000000000000000000 ) ) ;
#15783=ORIENTED_EDGE ( 'NONE', *, *, #32528, .F. ) ;
#15882=CARTESIAN_POINT ( 'NONE',  ( 10.00000000000000178, -46.01315789473684248, -5.916985404131818171 ) ) ;
#15903=AXIS2_PLACEMENT_3D ( 'NONE', #19731, #5074, #28196 ) ;
#15927=ORIENTED_EDGE ( 'NONE', *, *, #33702, .T. ) ;
#15944=FACE_OUTER_BOUND ( 'NONE', #120, .T. ) ;
#15967=LINE ( 'NONE', #31634, #21431 ) ;
#15987=ORIENTED_EDGE ( 'NONE', *, *, #2761, .T. ) ;
#15997=ORIENTED_EDGE ( 'NONE', *, *, #32162, .F. ) ;
#16010=VERTEX_POINT ( 'NONE', #49049 ) ;
#16035=VECTOR ( 'NONE', #13702, 1000.000000000000000 ) ;
#16078=DIRECTION ( 'NONE',  ( 1.000000000000000000, 0.000000000000000000, 0.000000000000000000 ) ) ;
#16093=VERTEX_POINT ( 'NONE', #17550 ) ;
#16150=EDGE_CURVE ( 'NONE', #11655, #28510, #46726, .T. ) ;
#16230=FACE_OUTER_BOUND ( 'NONE', #6724, .T. ) ;
#16238=CARTESIAN_POINT ( 'NONE',  ( 15.00000000000000000, -46.51315789473684248, 6.315789473684215949 ) ) ;
#16262=PLANE ( 'NONE',  #5287 ) ;
#16307=VERTEX_POINT ( 'NONE', #47000 ) ;
#16315=CARTESIAN_POINT ( 'NONE',  ( -14.49999999999999822, -46.01315789473684248, -5.916985404131817283 ) ) ;
#16339=DIRECTION ( 'NONE',  ( 0.000000000000000000, 0.000000000000000000, 1.000000000000000000 ) ) ;
#16369=EDGE_CURVE ( 'NONE', #32346, #44491, #23861, .T. ) ;
#16513=CIRCLE ( 'NONE', #27167, 5.000000000000000000 ) ;
#16599=VERTEX_POINT ( 'NONE', #47376 ) ;
#16636=DIRECTION ( 'NONE',  ( 0.000000000000000000, 0.000000000000000000, 1.000000000000000000 ) ) ;
#16644=CARTESIAN_POINT ( 'NONE',  ( 10.50000000000000178, -46.01315789473684248, 5.916985404131813731 ) ) ;
#16666=CARTESIAN_POINT ( 'NONE',  ( 15.00000000000000000, 12.98684210526315930, -19.37312575500899570 ) ) ;
#16696=AXIS2_PLACEMENT_3D ( 'NONE', #27687, #35407, #24102 ) ;
#16725=CARTESIAN_POINT ( 'NONE',  ( 10.50000000000000178, -46.01315789473684248, -5.916985404131818171 ) ) ;
#16825=CARTESIAN_POINT ( 'NONE',  ( 15.00000000000000000, 12.98684210526315930, 0.000000000000000000 ) ) ;
#17001=ORIENTED_EDGE ( 'NONE', *, *, #7113, .T. ) ;
#17016=DIRECTION ( 'NONE',  ( -6.938893903907233308E-16, 1.000000000000000000, 0.000000000000000000 ) ) ;
#17058=ORIENTED_EDGE ( 'NONE', *, *, #44355, .F. ) ;
#17085=FACE_OUTER_BOUND ( 'NONE', #21015, .T. ) ;
#17111=EDGE_CURVE ( 'NONE', #35640, #35926, #32492, .T. ) ;
#17118=CARTESIAN_POINT ( 'NONE',  ( 0.000000000000000000, 23.48684210526316107, -3.750000000000000000 ) ) ;
#17176=ORIENTED_EDGE ( 'NONE', *, *, #36041, .F. ) ;
#17189=AXIS2_PLACEMENT_3D ( 'NONE', #11558, #27206, #8470 ) ;
#17202=CARTESIAN_POINT ( 'NONE',  ( 0.000000000000000000, 13.98684210526316107, 0.000000000000000000 ) ) ;
#17208=AXIS2_PLACEMENT_3D ( 'NONE', #48170, #32330, #13059 ) ;
#17234=VECTOR ( 'NONE', #9626, 1000.000000000000000 ) ;
#17237=AXIS2_PLACEMENT_3D ( 'NONE', #36662, #5569, #8920 ) ;
#17275=DIRECTION ( 'NONE',  ( -6.765175596986472868E-16, 0.9749645535258953943, -0.2223603367690637489 ) ) ;
#17348=DIRECTION ( 'NONE',  ( 0.000000000000000000, 0.000000000000000000, -1.000000000000000000 ) ) ;
#17473=CIRCLE ( 'NONE', #43650, 0.5000000000000000000 ) ;
#17478=ORIENTED_EDGE ( 'NONE', *, *, #45007, .F. ) ;
#17520=CARTESIAN_POINT ( 'NONE',  ( 15.00000000000000000, 8.875661936878628921, -18.94832733001756253 ) ) ;
#17526=CARTESIAN_POINT ( 'NONE',  ( 0.000000000000000000, 13.98684210526316107, 0.000000000000000000 ) ) ;
#17532=ORIENTED_EDGE ( 'NONE', *, *, #26140, .T. ) ;
#17550=CARTESIAN_POINT ( 'NONE',  ( 9.999999999999996447, -34.54492135858216528, -5.000000000000000000 ) ) ;
#17565=EDGE_LOOP ( 'NONE', ( #27572, #44835, #7084 ) ) ;
#17587=CARTESIAN_POINT ( 'NONE',  ( 0.000000000000000000, 13.48684210526315930, 0.000000000000000000 ) ) ;
#17704=CYLINDRICAL_SURFACE ( 'NONE', #50233, 5.000000000000000000 ) ;
#17748=CARTESIAN_POINT ( 'NONE',  ( 0.000000000000000000, 23.48684210526316107, 0.000000000000000000 ) ) ;
#17761=EDGE_CURVE ( 'NONE', #11655, #37697, #20126, .T. ) ;
#17802=ORIENTED_EDGE ( 'NONE', *, *, #25959, .T. ) ;
#17826=CARTESIAN_POINT ( 'NONE',  ( -10.49999999999999467, -46.51315789473685669, 6.315789473684212396 ) ) ;
#17833=ADVANCED_FACE ( 'NONE', ( #4145 ), #12846, .T. ) ;
#17860=EDGE_CURVE ( 'NONE', #27491, #6443, #13343, .T. ) ;
#17958=DIRECTION ( 'NONE',  ( -0.000000000000000000, 0.9749645535258960605, -0.2223603367690608623 ) ) ;
#18020=CIRCLE ( 'NONE', #25398, 5.000000000000000000 ) ;
#18026=LINE ( 'NONE', #50036, #11518 ) ;
#18040=FACE_OUTER_BOUND ( 'NONE', #24214, .T. ) ;
#18052=EDGE_LOOP ( 'NONE', ( #11532, #895, #33028, #10074 ) ) ;
#18105=EDGE_LOOP ( 'NONE', ( #23898, #31101, #40640, #35582 ) ) ;
#18141=VERTEX_POINT ( 'NONE', #11783 ) ;
#18170=DIRECTION ( 'NONE',  ( -1.000000000000000000, -0.000000000000000000, -0.000000000000000000 ) ) ;
#18206=ORIENTED_EDGE ( 'NONE', *, *, #33064, .T. ) ;
#18212=FACE_OUTER_BOUND ( 'NONE', #20286, .T. ) ;
#18307=CARTESIAN_POINT ( 'NONE',  ( 14.49999999999999822, 12.87566193687862715, 19.86060803177194600 ) ) ;
#18419=FACE_OUTER_BOUND ( 'NONE', #171, .T. ) ;
#18471=ORIENTED_EDGE ( 'NONE', *, *, #2761, .F. ) ;
#18474=AXIS2_PLACEMENT_3D ( 'NONE', #48702, #44131, #24415 ) ;
#18497=CARTESIAN_POINT ( 'NONE',  ( -15.00199999999999712, -34.54492135858216528, 0.000000000000000000 ) ) ;
#18504=AXIS2_PLACEMENT_3D ( 'NONE', #10293, #7202, #6946 ) ;
#18517=LINE ( 'NONE', #17520, #33190 ) ;
#18531=CARTESIAN_POINT ( 'NONE',  ( 0.000000000000000000, 23.48684210526316107, 0.000000000000000000 ) ) ;
#18584=DIRECTION ( 'NONE',  ( 0.000000000000000000, 0.000000000000000000, -1.000000000000000000 ) ) ;
#18596=CARTESIAN_POINT ( 'NONE',  ( 14.49999999999999822, 12.98684210526315930, 19.37312575500900280 ) ) ;
#18599=AXIS2_PLACEMENT_3D ( 'NONE', #15616, #34883, #27422 ) ;
#18607=ADVANCED_FACE ( 'NONE', ( #28825 ), #20900, .F. ) ;
#18673=CARTESIAN_POINT ( 'NONE',  ( 0.000000000000000000, 13.98684210526316107, -4.250000000000000000 ) ) ;
#18674=DIRECTION ( 'NONE',  ( 0.000000000000000000, -0.000000000000000000, 1.000000000000000000 ) ) ;
#18790=DIRECTION ( 'NONE',  ( 0.000000000000000000, 0.000000000000000000, 1.000000000000000000 ) ) ;
#18797=DIRECTION ( 'NONE',  ( 0.000000000000000000, 1.000000000000000000, 1.387778780781444413E-14 ) ) ;
#18804=DIRECTION ( 'NONE',  ( 0.000000000000000000, 0.2223603367690619725, -0.9749645535258958384 ) ) ;
#18825=ORIENTED_EDGE ( 'NONE', *, *, #4241, .F. ) ;
#18826=CARTESIAN_POINT ( 'NONE',  ( 14.49999999999999822, -3.557843729863134463, -15.59977635401528850 ) ) ;
#18832=DIRECTION ( 'NONE',  ( 0.000000000000000000, 0.000000000000000000, 1.000000000000000000 ) ) ;
#18907=DIRECTION ( 'NONE',  ( 0.000000000000000000, 0.000000000000000000, -1.000000000000000000 ) ) ;
#18997=DIRECTION ( 'NONE',  ( -1.000000000000000000, 0.000000000000000000, 0.000000000000000000 ) ) ;
#18999=CARTESIAN_POINT ( 'NONE',  ( 6.123233995736766282E-16, 23.48684210526316107, 5.000000000000000000 ) ) ;
#19007=EDGE_CURVE ( 'NONE', #37345, #44491, #32881, .T. ) ;
#19061=AXIS2_PLACEMENT_3D ( 'NONE', #17748, #21858, #6204 ) ;
#19091=DIRECTION ( 'NONE',  ( 0.000000000000000000, -0.000000000000000000, 1.000000000000000000 ) ) ;
#19117=ORIENTED_EDGE ( 'NONE', *, *, #23784, .T. ) ;
#19180=FACE_OUTER_BOUND ( 'NONE', #8082, .T. ) ;
#19188=CARTESIAN_POINT ( 'NONE',  ( -10.49999999999999467, -46.12433806312137108, -6.404467680894765813 ) ) ;
#19208=DIRECTION ( 'NONE',  ( 0.000000000000000000, 8.673617379884027583E-15, -1.000000000000000000 ) ) ;
#19221=VERTEX_POINT ( 'NONE', #35672 ) ;
#19237=FACE_OUTER_BOUND ( 'NONE', #23760, .T. ) ;
#19365=AXIS2_PLACEMENT_3D ( 'NONE', #15301, #38908, #24454 ) ;
#19373=AXIS2_PLACEMENT_3D ( 'NONE', #42842, #39028, #26707 ) ;
#19420=DIRECTION ( 'NONE',  ( 0.000000000000000000, -0.9749645535258955054, 0.2223603367690637767 ) ) ;
#19453=ORIENTED_EDGE ( 'NONE', *, *, #39960, .T. ) ;
#19459=VECTOR ( 'NONE', #43255, 1000.000000000000000 ) ;
#19476=DIRECTION ( 'NONE',  ( 0.000000000000000000, 0.000000000000000000, -1.000000000000000000 ) ) ;
#19477=ORIENTED_EDGE ( 'NONE', *, *, #5606, .T. ) ;
#19567=EDGE_LOOP ( 'NONE', ( #19822, #29399, #12002, #6187 ) ) ;
#19609=AXIS2_PLACEMENT_3D ( 'NONE', #13606, #6166, #22312 ) ;
#19725=VECTOR ( 'NONE', #7733, 1000.000000000000000 ) ;
#19731=CARTESIAN_POINT ( 'NONE',  ( 14.49999999999999822, 12.98684210526315930, 19.37312575500900280 ) ) ;
#19732=DIRECTION ( 'NONE',  ( 0.000000000000000000, 0.000000000000000000, -1.000000000000000000 ) ) ;
#19741=ORIENTED_EDGE ( 'NONE', *, *, #20236, .F. ) ;
#19764=VERTEX_POINT ( 'NONE', #12997 ) ;
#19777=CARTESIAN_POINT ( 'NONE',  ( 0.000000000000000000, 23.48684210526316107, 0.000000000000000000 ) ) ;
#19792=VECTOR ( 'NONE', #29091, 1000.000000000000000 ) ;
#19796=CARTESIAN_POINT ( 'NONE',  ( 10.50000000000000178, -46.01315789473684248, 5.916985404131813731 ) ) ;
#19817=ORIENTED_EDGE ( 'NONE', *, *, #30537, .T. ) ;
#19822=ORIENTED_EDGE ( 'NONE', *, *, #9570, .T. ) ;
#19859=CYLINDRICAL_SURFACE ( 'NONE', #49112, 0.4999999999999992228 ) ;
#19899=ORIENTED_EDGE ( 'NONE', *, *, #7062, .T. ) ;
#19920=DIRECTION ( 'NONE',  ( 0.000000000000000000, -0.2223603367690619725, 0.9749645535258958384 ) ) ;
#19931=EDGE_LOOP ( 'NONE', ( #21666, #47687, #39202, #28408, #3785, #45626, #28744, #46957 ) ) ;
#20079=LINE ( 'NONE', #4431, #7910 ) ;
#20114=DIRECTION ( 'NONE',  ( 0.000000000000000000, -0.000000000000000000, 1.000000000000000000 ) ) ;
#20118=LINE ( 'NONE', #23725, #45030 ) ;
#20126=CIRCLE ( 'NONE', #37346, 0.4999999999999997224 ) ;
#20146=ORIENTED_EDGE ( 'NONE', *, *, #3241, .T. ) ;
#20206=EDGE_CURVE ( 'NONE', #10704, #28357, #33233, .T. ) ;
#20236=EDGE_CURVE ( 'NONE', #27759, #42182, #21656, .T. ) ;
#20256=DIRECTION ( 'NONE',  ( -1.000000000000000000, 0.000000000000000000, 0.000000000000000000 ) ) ;
#20269=ADVANCED_FACE ( 'NONE', ( #29866 ), #32978, .T. ) ;
#20286=EDGE_LOOP ( 'NONE', ( #17532, #23944, #7809, #39762 ) ) ;
#20304=VERTEX_POINT ( 'NONE', #41917 ) ;
#20367=FACE_OUTER_BOUND ( 'NONE', #11142, .T. ) ;
#20403=VECTOR ( 'NONE', #40686, 1000.000000000000114 ) ;
#20443=ADVANCED_FACE ( 'NONE', ( #37842 ), #34232, .T. ) ;
#20536=VERTEX_POINT ( 'NONE', #24455 ) ;
#20570=CARTESIAN_POINT ( 'NONE',  ( 0.000000000000000000, 13.48684210526315930, -4.250000000000000000 ) ) ;
#20587=DIRECTION ( 'NONE',  ( 1.000000000000000000, -0.000000000000000000, -0.000000000000000000 ) ) ;
#20644=FACE_OUTER_BOUND ( 'NONE', #34403, .T. ) ;
#20686=ORIENTED_EDGE ( 'NONE', *, *, #7113, .F. ) ;
#20691=CARTESIAN_POINT ( 'NONE',  ( 10.01251772323701772, 8.486842105263161073, 18.46084505325461578 ) ) ;
#20701=VERTEX_POINT ( 'NONE', #18999 ) ;
#20728=APPLICATION_CONTEXT ( 'automotive_design' ) ;
#20745=CARTESIAN_POINT ( 'NONE',  ( 5.204748896376250699E-16, 13.98684210526316107, 4.250000000000000000 ) ) ;
#20758=CIRCLE ( 'NONE', #26592, 0.5000000000000004441 ) ;
#20896=CARTESIAN_POINT ( 'NONE',  ( 10.49999999999996092, 13.59802227364768967, -19.51251772323705325 ) ) ;
#20900=TOROIDAL_SURFACE ( 'NONE', #41376, 4.250000000000000000, 0.5000000000000000000 ) ;
#20945=CARTESIAN_POINT ( 'NONE',  ( 0.000000000000000000, 28.48684210526315752, 0.000000000000000000 ) ) ;
#21006=AXIS2_PLACEMENT_3D ( 'NONE', #16238, #599, #31899 ) ;
#21015=EDGE_LOOP ( 'NONE', ( #24682, #4256, #11227 ) ) ;
#21050=PRODUCT_CONTEXT ( 'NONE', #48559, 'mechanical' ) ;
#21124=ORIENTED_EDGE ( 'NONE', *, *, #44448, .F. ) ;
#21164=FACE_OUTER_BOUND ( 'NONE', #12205, .T. ) ;
#21280=ORIENTED_EDGE ( 'NONE', *, *, #17111, .F. ) ;
#21290=AXIS2_PLACEMENT_3D ( 'NONE', #25290, #6306, #18584 ) ;
#21319=DIRECTION ( 'NONE',  ( 1.000000000000000000, -0.000000000000000000, 0.000000000000000000 ) ) ;
#21368=DIRECTION ( 'NONE',  ( 0.000000000000000000, 0.000000000000000000, -1.000000000000000000 ) ) ;
#21419=CARTESIAN_POINT ( 'NONE',  ( 10.01251772323701772, 8.486842105263161073, 18.46084505325461578 ) ) ;
#21431=VECTOR ( 'NONE', #26496, 1000.000000000000000 ) ;
#21467=EDGE_LOOP ( 'NONE', ( #3663, #26686, #15654, #3932, #7922 ) ) ;
#21481=AXIS2_PLACEMENT_3D ( 'NONE', #38080, #30371, #18797 ) ;
#21519=CIRCLE ( 'NONE', #19061, 3.750000000000000000 ) ;
#21525=EDGE_CURVE ( 'NONE', #16093, #6443, #38183, .T. ) ;
#21540=CIRCLE ( 'NONE', #13333, 0.5000000000000004441 ) ;
#21547=ORIENTED_EDGE ( 'NONE', *, *, #23304, .F. ) ;
#21554=CARTESIAN_POINT ( 'NONE',  ( 14.49999999999999822, 12.87566193687862715, -19.86060803177194956 ) ) ;
#21563=AXIS2_PLACEMENT_3D ( 'NONE', #39200, #31499, #43527 ) ;
#21588=CARTESIAN_POINT ( 'NONE',  ( 10.49999999999996447, 8.875661936878628921, -18.94832733001756253 ) ) ;
#21609=CIRCLE ( 'NONE', #46180, 0.5000000000000004441 ) ;
#21613=CARTESIAN_POINT ( 'NONE',  ( 14.49999999999999822, -46.51315789473684248, -5.916985404131818171 ) ) ;
#21656=LINE ( 'NONE', #25768, #16035 ) ;
#21666=ORIENTED_EDGE ( 'NONE', *, *, #32494, .T. ) ;
#21667=CARTESIAN_POINT ( 'NONE',  ( 14.49999999999999822, 12.98684210526315930, -19.37312575500900280 ) ) ;
#21711=FACE_OUTER_BOUND ( 'NONE', #27334, .T. ) ;
#21725=ADVANCED_FACE ( 'NONE', ( #35957 ), #28498, .T. ) ;
#21785=ORIENTED_EDGE ( 'NONE', *, *, #13439, .F. ) ;
#21818=ORIENTED_EDGE ( 'NONE', *, *, #33759, .T. ) ;
#21858=DIRECTION ( 'NONE',  ( 0.000000000000000000, 1.000000000000000000, 0.000000000000000000 ) ) ;
#21943=DIRECTION ( 'NONE',  ( 0.000000000000000000, -1.000000000000000000, 0.000000000000000000 ) ) ;
#21956=CARTESIAN_POINT ( 'NONE',  ( 14.49999999999999822, 12.98684210526315930, -19.37312575500900280 ) ) ;
#22025=DIRECTION ( 'NONE',  ( -1.000000000000000000, 0.000000000000000000, 1.387778780781444413E-14 ) ) ;
#22043=DIRECTION ( 'NONE',  ( -1.000000000000000000, 0.000000000000000000, 0.000000000000000000 ) ) ;
#22049=CARTESIAN_POINT ( 'NONE',  ( 15.00000000000000000, -46.51315789473684248, -6.315789473684215949 ) ) ;
#22090=CARTESIAN_POINT ( 'NONE',  ( 10.50000000000000178, -46.01315789473684248, 5.916985404131814619 ) ) ;
#22202=CARTESIAN_POINT ( 'NONE',  ( 9.999999999999964473, 8.486842105263161073, -18.38522261288946780 ) ) ;
#22312=DIRECTION ( 'NONE',  ( 0.000000000000000000, 0.000000000000000000, 1.000000000000000000 ) ) ;
#22320=MANIFOLD_SOLID_BREP ( 'Fillet1', #39230 ) ;
#22339=VECTOR ( 'NONE', #19476, 1000.000000000000000 ) ;
#22359=ORIENTED_EDGE ( 'NONE', *, *, #47440, .T. ) ;
#22404=CARTESIAN_POINT ( 'NONE',  ( -14.49999999999999822, 12.98684210526315930, 19.87312575500899925 ) ) ;
#22432=VECTOR ( 'NONE', #24015, 1000.000000000000000 ) ;
#22461=CARTESIAN_POINT ( 'NONE',  ( -15.00199999999999712, -34.54492135858216528, -5.000000000000000000 ) ) ;
#22576=ORIENTED_EDGE ( 'NONE', *, *, #40015, .T. ) ;
#22589=AXIS2_PLACEMENT_3D ( 'NONE', #29815, #10323, #28810 ) ;
#22613=CIRCLE ( 'NONE', #46350, 0.5000000000000004441 ) ;
#22686=ADVANCED_FACE ( 'NONE', ( #19180 ), #31266, .F. ) ;
#22716=ORIENTED_EDGE ( 'NONE', *, *, #5606, .F. ) ;
#22717=CARTESIAN_POINT ( 'NONE',  ( -10.25676241992221449, 8.638513918217336496, 18.89424093979656405 ) ) ;
#22901=CIRCLE ( 'NONE', #34381, 0.4999999999999992228 ) ;
#22921=CYLINDRICAL_SURFACE ( 'NONE', #27986, 0.4999999999999997224 ) ;
#22949=DIRECTION ( 'NONE',  ( 0.000000000000000000, 1.000000000000000000, 0.000000000000000000 ) ) ;
#22953=DIRECTION ( 'NONE',  ( 0.000000000000000000, 0.000000000000000000, 1.000000000000000000 ) ) ;
#22962=ORIENTED_EDGE ( 'NONE', *, *, #28054, .F. ) ;
#23020=ORIENTED_EDGE ( 'NONE', *, *, #3855, .T. ) ;
#23050=EDGE_CURVE ( 'NONE', #44491, #10704, #43897, .T. ) ;
#23109=LINE ( 'NONE', #7479, #11169 ) ;
#23110=VERTEX_POINT ( 'NONE', #973 ) ;
#23196=EDGE_CURVE ( 'NONE', #44491, #609, #9915, .T. ) ;
#23205=CARTESIAN_POINT ( 'NONE',  ( -10.50000000000003730, 13.59802227364767546, -19.51251772323704969 ) ) ;
#23259=CARTESIAN_POINT ( 'NONE',  ( -14.49999999999999822, -46.40197772635230677, 5.828307196921268307 ) ) ;
#23262=AXIS2_PLACEMENT_3D ( 'NONE', #48635, #25097, #1496 ) ;
#23295=ORIENTED_EDGE ( 'NONE', *, *, #24735, .T. ) ;
#23304=EDGE_CURVE ( 'NONE', #7866, #1161, #11437, .T. ) ;
#23311=LINE ( 'NONE', #38986, #29835 ) ;
#23317=EDGE_CURVE ( 'NONE', #28357, #11655, #38398, .T. ) ;
#23322=EDGE_CURVE ( 'NONE', #27491, #20536, #39865, .T. ) ;
#23339=CARTESIAN_POINT ( 'NONE',  ( -10.49999999999999467, -46.01315789473684248, -5.916985404131818171 ) ) ;
#23348=CARTESIAN_POINT ( 'NONE',  ( -15.00000000000000000, -46.01315789473684248, 5.916985404131813731 ) ) ;
#23351=VECTOR ( 'NONE', #12641, 1000.000000000000114 ) ;
#23352=VECTOR ( 'NONE', #5908, 1000.000000000000000 ) ;
#23384=CARTESIAN_POINT ( 'NONE',  ( 9.999999999999998224, 8.486842105263161073, -25.00000000000000000 ) ) ;
#23409=LINE ( 'NONE', #15699, #44996 ) ;
#23444=AXIS2_PLACEMENT_3D ( 'NONE', #31522, #15356, #18674 ) ;
#23477=CYLINDRICAL_SURFACE ( 'NONE', #6530, 3.750000000000000000 ) ;
#23498=VERTEX_POINT ( 'NONE', #33659 ) ;
#23501=EDGE_CURVE ( 'NONE', #12400, #18141, #23109, .T. ) ;
#23531=ADVANCED_FACE ( 'NONE', ( #41602 ), #26960, .T. ) ;
#23543=CARTESIAN_POINT ( 'NONE',  ( 10.50000000000000178, -46.01315789473684248, -25.00000000000000000 ) ) ;
#23596=DIRECTION ( 'NONE',  ( 0.000000000000000000, 0.000000000000000000, -1.000000000000000000 ) ) ;
#23637=LINE ( 'NONE', #23384, #4835 ) ;
#23640=AXIS2_PLACEMENT_3D ( 'NONE', #32676, #48273, #28824 ) ;
#23725=CARTESIAN_POINT ( 'NONE',  ( 10.50000000000000178, -46.51315789473684248, 6.315789473684215061 ) ) ;
#23760=EDGE_LOOP ( 'NONE', ( #10327, #14785, #1845, #48649 ) ) ;
#23784=EDGE_CURVE ( 'NONE', #16307, #10704, #13649, .T. ) ;
#23788=FACE_OUTER_BOUND ( 'NONE', #28959, .T. ) ;
#23833=DIRECTION ( 'NONE',  ( -0.000000000000000000, -0.000000000000000000, -1.000000000000000000 ) ) ;
#23842=FACE_OUTER_BOUND ( 'NONE', #8402, .T. ) ;
#23861=CIRCLE ( 'NONE', #30407, 0.5000000000000004441 ) ;
#23898=ORIENTED_EDGE ( 'NONE', *, *, #38861, .F. ) ;
#23925=ORIENTED_EDGE ( 'NONE', *, *, #37750, .F. ) ;
#23944=ORIENTED_EDGE ( 'NONE', *, *, #28633, .T. ) ;
#23954=ORIENTED_EDGE ( 'NONE', *, *, #33677, .T. ) ;
#23963=EDGE_LOOP ( 'NONE', ( #1272, #20146, #10297 ) ) ;
#23973=CARTESIAN_POINT ( 'NONE',  ( 15.00000000000000000, -46.51315789473684248, -6.315789473684215949 ) ) ;
#23983=CARTESIAN_POINT ( 'NONE',  ( 10.49999999999996092, 13.48684210526315574, -20.00000000000000000 ) ) ;
#23996=DIRECTION ( 'NONE',  ( 0.000000000000000000, 0.2223603367690656640, 0.9749645535258950613 ) ) ;
#23998=CARTESIAN_POINT ( 'NONE',  ( 10.49999999999996447, 8.875661936878628921, -18.94832733001756253 ) ) ;
#24015=DIRECTION ( 'NONE',  ( -0.000000000000000000, -0.000000000000000000, 1.000000000000000000 ) ) ;
#24081=AXIS2_PLACEMENT_3D ( 'NONE', #8941, #11785, #39245 ) ;
#24098=DIRECTION ( 'NONE',  ( 0.000000000000000000, 1.000000000000000000, 0.000000000000000000 ) ) ;
#24102=DIRECTION ( 'NONE',  ( 3.469446951953616950E-15, 0.000000000000000000, -1.000000000000000000 ) ) ;
#24156=CARTESIAN_POINT ( 'NONE',  ( -14.49999999999999822, -46.51315789473684248, 6.315789473684215949 ) ) ;
#24214=EDGE_LOOP ( 'NONE', ( #23295, #26528, #46555, #21547 ) ) ;
#24279=DIRECTION ( 'NONE',  ( 3.469446951953616950E-15, 0.000000000000000000, 1.000000000000000000 ) ) ;
#24295=VECTOR ( 'NONE', #20587, 1000.000000000000000 ) ;
#24326=EDGE_CURVE ( 'NONE', #20536, #27491, #34886, .T. ) ;
#24365=CARTESIAN_POINT ( 'NONE',  ( -14.49999999999999822, -46.51315789473684248, -6.315789473684215949 ) ) ;
#24408=DIRECTION ( 'NONE',  ( -0.000000000000000000, -1.000000000000000000, -0.000000000000000000 ) ) ;
#24415=DIRECTION ( 'NONE',  ( -1.000000000000000000, 0.000000000000000000, 0.000000000000000000 ) ) ;
#24454=DIRECTION ( 'NONE',  ( 6.938893903907232322E-16, -1.000000000000000000, 0.000000000000000000 ) ) ;
#24455=CARTESIAN_POINT ( 'NONE',  ( -10.00000000000000355, -34.54492135858216528, -5.000000000000000000 ) ) ;
#24463=CARTESIAN_POINT ( 'NONE',  ( 14.49999999999999822, 12.98684210526315930, 19.37312575500900280 ) ) ;
#24517=ORIENTED_EDGE ( 'NONE', *, *, #36920, .F. ) ;
#24519=CARTESIAN_POINT ( 'NONE',  ( 15.00000000000000000, 12.98684210526315752, 19.87312575500900280 ) ) ;
#24526=AXIS2_PLACEMENT_3D ( 'NONE', #10272, #5654, #37496 ) ;
#24549=CARTESIAN_POINT ( 'NONE',  ( 15.00000000000000000, -46.12433806312137108, 6.404467680894761372 ) ) ;
#24578=ORIENTED_EDGE ( 'NONE', *, *, #592, .T. ) ;
#24579=EDGE_CURVE ( 'NONE', #46782, #35640, #38917, .T. ) ;
#24586=DIRECTION ( 'NONE',  ( 0.000000000000000000, 0.000000000000000000, -1.000000000000000000 ) ) ;
#24669=VERTEX_POINT ( 'NONE', #6516 ) ;
#24682=ORIENTED_EDGE ( 'NONE', *, *, #25208, .T. ) ;
#24708=VECTOR ( 'NONE', #34222, 1000.000000000000114 ) ;
#24717=CARTESIAN_POINT ( 'NONE',  ( 0.000000000000000000, 23.48684210526316107, -3.750000000000000000 ) ) ;
#24735=EDGE_CURVE ( 'NONE', #7866, #40121, #40464, .T. ) ;
#24749=AXIS2_PLACEMENT_3D ( 'NONE', #18826, #11154, #26801 ) ;
#24767=EDGE_LOOP ( 'NONE', ( #46817, #29021, #9406, #13871 ) ) ;
#24819=ORIENTED_EDGE ( 'NONE', *, *, #37750, .T. ) ;
#24837=CARTESIAN_POINT ( 'NONE',  ( -10.25676241992221449, 8.638513918217338272, -18.89424093979656760 ) ) ;
#24880=DIRECTION ( 'NONE',  ( -1.000000000000000000, 0.000000000000000000, 0.000000000000000000 ) ) ;
#24893=EDGE_LOOP ( 'NONE', ( #7829, #4487, #44338, #47801 ) ) ;
#24926=EDGE_CURVE ( 'NONE', #43437, #46782, #7806, .T. ) ;
#24944=VERTEX_POINT ( 'NONE', #24717 ) ;
#24959=DIRECTION ( 'NONE',  ( 0.000000000000000000, -0.2223603367690689669, 0.9749645535258942841 ) ) ;
#24978=VECTOR ( 'NONE', #41875, 1000.000000000000000 ) ;
#25079=EDGE_CURVE ( 'NONE', #12918, #23110, #2933, .T. ) ;
#25097=DIRECTION ( 'NONE',  ( -0.000000000000000000, 1.000000000000000000, 0.000000000000000000 ) ) ;
#25127=DIRECTION ( 'NONE',  ( 0.000000000000000000, 0.000000000000000000, 1.000000000000000000 ) ) ;
#25133=DIRECTION ( 'NONE',  ( 1.000000000000000000, -0.000000000000000000, -0.000000000000000000 ) ) ;
#25140=ORIENTED_EDGE ( 'NONE', *, *, #7478, .F. ) ;
#25142=CARTESIAN_POINT ( 'NONE',  ( -14.49999999999999822, -46.01315789473684248, 5.916985404131813731 ) ) ;
#25192=ORIENTED_EDGE ( 'NONE', *, *, #46532, .F. ) ;
#25208=EDGE_CURVE ( 'NONE', #19221, #5824, #4458, .T. ) ;
#25209=CARTESIAN_POINT ( 'NONE',  ( -10.00000000000003375, 8.486842105263161073, -18.38522261288946780 ) ) ;
#25233=EDGE_CURVE ( 'NONE', #16307, #16010, #23311, .T. ) ;
#25290=CARTESIAN_POINT ( 'NONE',  ( -10.49999999999999467, -46.01315789473684248, 5.916985404131813731 ) ) ;
#25296=ADVANCED_FACE ( 'NONE', ( #4075 ), #9431, .T. ) ;
#25322=FACE_OUTER_BOUND ( 'NONE', #2968, .T. ) ;
#25344=ADVANCED_FACE ( 'NONE', ( #13774 ), #33309, .T. ) ;
#25360=CARTESIAN_POINT ( 'NONE',  ( 0.000000000000000000, 13.98684210526316107, -3.750000000000000000 ) ) ;
#25371=VECTOR ( 'NONE', #39639, 1000.000000000000000 ) ;
#25398=AXIS2_PLACEMENT_3D ( 'NONE', #50096, #22949, #49596 ) ;
#25468=ORIENTED_EDGE ( 'NONE', *, *, #44448, .T. ) ;
#25486=CARTESIAN_POINT ( 'NONE',  ( 10.50000000000000178, -46.01315789473684248, -5.916985404131818171 ) ) ;
#25504=CARTESIAN_POINT ( 'NONE',  ( -10.50000000000003375, 8.875661936878630698, 18.94832733001756253 ) ) ;
#25506=ORIENTED_EDGE ( 'NONE', *, *, #41494, .F. ) ;
#25571=CYLINDRICAL_SURFACE ( 'NONE', #6954, 0.5000000000000004441 ) ;
#25647=AXIS2_PLACEMENT_3D ( 'NONE', #12093, #8245, #4650 ) ;
#25768=CARTESIAN_POINT ( 'NONE',  ( 15.00000000000000000, -46.12433806312137108, 6.404467680894761372 ) ) ;
#25775=DIRECTION ( 'NONE',  ( 1.000000000000000000, 0.000000000000000000, -0.000000000000000000 ) ) ;
#25815=LINE ( 'NONE', #22461, #7040 ) ;
#25817=EDGE_CURVE ( 'NONE', #42182, #3066, #29884, .T. ) ;
#25886=CYLINDRICAL_SURFACE ( 'NONE', #30239, 5.000000000000000000 ) ;
#25894=DIRECTION ( 'NONE',  ( -0.000000000000000000, 0.000000000000000000, -1.000000000000000000 ) ) ;
#25920=CARTESIAN_POINT ( 'NONE',  ( 0.000000000000000000, 28.48684210526315752, 0.000000000000000000 ) ) ;
#25938=CARTESIAN_POINT ( 'NONE',  ( -14.49999999999999822, -46.01315789473684248, 5.916985404131813731 ) ) ;
#25947=LINE ( 'NONE', #10530, #4021 ) ;
#25959=EDGE_CURVE ( 'NONE', #47807, #9479, #28231, .T. ) ;
#26003=ADVANCED_FACE ( 'NONE', ( #12407, #28061 ), #16262, .F. ) ;
#26012=CARTESIAN_POINT ( 'NONE',  ( 15.00000000000000000, -46.01315789473684248, -5.916985404131818171 ) ) ;
#26050=LINE ( 'NONE', #14229, #26132 ) ;
#26074=CARTESIAN_POINT ( 'NONE',  ( 15.00000000000000000, 12.87566193687862004, 19.86060803177194956 ) ) ;
#26075=ORIENTED_EDGE ( 'NONE', *, *, #23196, .F. ) ;
#26132=VECTOR ( 'NONE', #10399, 1000.000000000000000 ) ;
#26140=EDGE_CURVE ( 'NONE', #39173, #8236, #2857, .T. ) ;
#26148=FACE_OUTER_BOUND ( 'NONE', #34740, .T. ) ;
#26162=EDGE_CURVE ( 'NONE', #28181, #23498, #18517, .T. ) ;
#26179=DIRECTION ( 'NONE',  ( 0.000000000000000000, -1.000000000000000000, 1.734723475976805517E-15 ) ) ;
#26276=AXIS2_PLACEMENT_3D ( 'NONE', #42765, #207, #43027 ) ;
#26307=DIRECTION ( 'NONE',  ( 0.000000000000000000, 1.000000000000000000, 0.000000000000000000 ) ) ;
#26357=AXIS2_PLACEMENT_3D ( 'NONE', #18531, #30102, #29844 ) ;
#26378=CARTESIAN_POINT ( 'NONE',  ( -9.999999999999998224, 8.486842105263161073, 18.34680996553531784 ) ) ;
#26405=AXIS2_PLACEMENT_3D ( 'NONE', #3180, #30662, #18832 ) ;
#26422=DIRECTION ( 'NONE',  ( 0.000000000000000000, 1.734723475976805319E-15, 1.000000000000000000 ) ) ;
#26472=DIRECTION ( 'NONE',  ( 0.000000000000000000, 0.000000000000000000, -1.000000000000000000 ) ) ;
#26496=DIRECTION ( 'NONE',  ( 6.765175596986472868E-16, -0.9749645535258953943, -0.2223603367690637489 ) ) ;
#26499=ORIENTED_EDGE ( 'NONE', *, *, #15503, .F. ) ;
#26528=ORIENTED_EDGE ( 'NONE', *, *, #38369, .F. ) ;
#26565=PRODUCT ( 'tire holder', 'tire holder', '', ( #21050 ) ) ;
#26592=AXIS2_PLACEMENT_3D ( 'NONE', #45587, #6871, #18907 ) ;
#26622=DIRECTION ( 'NONE',  ( 0.000000000000000000, 1.000000000000000000, 0.000000000000000000 ) ) ;
#26666=CARTESIAN_POINT ( 'NONE',  ( -9.999999999999998224, 8.486842105263161073, -18.34680996553531784 ) ) ;
#26686=ORIENTED_EDGE ( 'NONE', *, *, #32682, .F. ) ;
#26707=DIRECTION ( 'NONE',  ( 0.000000000000000000, 0.000000000000000000, -1.000000000000000000 ) ) ;
#26750=DIRECTION ( 'NONE',  ( -0.000000000000000000, -1.000000000000000000, -0.000000000000000000 ) ) ;
#26781=CARTESIAN_POINT ( 'NONE',  ( -10.49999999999999467, -46.40197772635232099, 5.828307196921264755 ) ) ;
#26801=DIRECTION ( 'NONE',  ( 0.000000000000000000, 0.2223603367690632493, 0.9749645535258955054 ) ) ;
#26814=ADVANCED_FACE ( 'NONE', ( #29652 ), #41193, .T. ) ;
#26818=DIRECTION ( 'NONE',  ( -1.000000000000000000, 0.000000000000000000, 0.000000000000000000 ) ) ;
#26821=ORIENTED_EDGE ( 'NONE', *, *, #8416, .F. ) ;
#26840=VERTEX_POINT ( 'NONE', #2697 ) ;
#26886=DIRECTION ( 'NONE',  ( 0.000000000000000000, -1.000000000000000000, 8.673617379884027583E-15 ) ) ;
#26960=CYLINDRICAL_SURFACE ( 'NONE', #32503, 5.000000000000000000 ) ;
#26971=CIRCLE ( 'NONE', #36011, 0.5000000000000004441 ) ;
#27007=DIRECTION ( 'NONE',  ( -0.000000000000000000, -0.000000000000000000, 1.000000000000000000 ) ) ;
#27026=CARTESIAN_POINT ( 'NONE',  ( 10.50000000000000178, -46.40197772635230677, 5.828307196921267419 ) ) ;
#27039=SHAPE_REPRESENTATION_RELATIONSHIP ( 'NONE' , 'NONE' ,  #35275, #27107 ) ;
#27076=AXIS2_PLACEMENT_3D ( 'NONE', #42127, #38318, #41386 ) ;
#27095=CARTESIAN_POINT ( 'NONE',  ( 10.50000000000000178, -46.12433806312137108, -6.404467680894765813 ) ) ;
#27107=ADVANCED_BREP_SHAPE_REPRESENTATION ( '', ( #22320, #45486 ), #13533 ) ;
#27117=DIRECTION ( 'NONE',  ( 0.000000000000000000, -0.9749645535258955054, -0.2223603367690637767 ) ) ;
#27167=AXIS2_PLACEMENT_3D ( 'NONE', #49418, #26622, #2752 ) ;
#27184=DIRECTION ( 'NONE',  ( 0.000000000000000000, -1.000000000000000000, 0.000000000000000000 ) ) ;
#27206=DIRECTION ( 'NONE',  ( -1.000000000000000000, 0.000000000000000000, 0.000000000000000000 ) ) ;
#27270=ORIENTED_EDGE ( 'NONE', *, *, #41494, .T. ) ;
#27334=EDGE_LOOP ( 'NONE', ( #47929, #19477, #14739, #26075 ) ) ;
#27337=DIRECTION ( 'NONE',  ( 1.000000000000000000, -0.000000000000000000, -0.000000000000000000 ) ) ;
#27360=LINE ( 'NONE', #15319, #19459 ) ;
#27415=ADVANCED_FACE ( 'NONE', ( #16230 ), #35236, .T. ) ;
#27422=DIRECTION ( 'NONE',  ( 0.000000000000000000, 0.000000000000000000, 1.000000000000000000 ) ) ;
#27488=DIRECTION ( 'NONE',  ( 0.000000000000000000, 0.000000000000000000, -1.000000000000000000 ) ) ;
#27491=VERTEX_POINT ( 'NONE', #80 ) ;
#27572=ORIENTED_EDGE ( 'NONE', *, *, #38408, .T. ) ;
#27573=ORIENTED_EDGE ( 'NONE', *, *, #16369, .T. ) ;
#27622=EDGE_LOOP ( 'NONE', ( #32517, #19741, #15783, #50519 ) ) ;
#27687=CARTESIAN_POINT ( 'NONE',  ( -10.49999999999999467, -46.01315789473684248, -5.916985404131817283 ) ) ;
#27698=ADVANCED_FACE ( 'NONE', ( #42340, #19237 ), #34407, .F. ) ;
#27746=CARTESIAN_POINT ( 'NONE',  ( 14.49999999999999822, -46.01315789473684248, -5.916985404131817283 ) ) ;
#27759=VERTEX_POINT ( 'NONE', #45658 ) ;
#27825=PLANE ( 'NONE',  #29787 ) ;
#27829=ORIENTED_EDGE ( 'NONE', *, *, #19007, .T. ) ;
#27855=EDGE_LOOP ( 'NONE', ( #36604, #17802 ) ) ;
#27864=ORIENTED_EDGE ( 'NONE', *, *, #16150, .F. ) ;
#27986=AXIS2_PLACEMENT_3D ( 'NONE', #27026, #7798, #18804 ) ;
#28003=ADVANCED_FACE ( 'NONE', ( #32840 ), #9717, .T. ) ;
#28026=CIRCLE ( 'NONE', #4260, 0.4999999999999996114 ) ;
#28054=EDGE_CURVE ( 'NONE', #8236, #49488, #22613, .T. ) ;
#28061=FACE_OUTER_BOUND ( 'NONE', #42335, .T. ) ;
#28117=DIRECTION ( 'NONE',  ( 0.000000000000000000, 1.000000000000000000, -0.000000000000000000 ) ) ;
#28134=CARTESIAN_POINT ( 'NONE',  ( 10.01251772323701772, 8.486842105263161073, 18.46084505325461578 ) ) ;
#28171=ORIENTED_EDGE ( 'NONE', *, *, #30537, .F. ) ;
#28173=DIRECTION ( 'NONE',  ( 0.000000000000000000, 0.9749645535258950613, -0.2223603367690656918 ) ) ;
#28181=VERTEX_POINT ( 'NONE', #23998 ) ;
#28186=DIRECTION ( 'NONE',  ( 0.000000000000000000, 0.000000000000000000, 1.000000000000000000 ) ) ;
#28196=DIRECTION ( 'NONE',  ( 0.000000000000000000, 0.000000000000000000, -1.000000000000000000 ) ) ;
#28222=DIRECTION ( 'NONE',  ( 0.000000000000000000, 0.000000000000000000, 1.000000000000000000 ) ) ;
#28227=PLANE ( 'NONE',  #38879 ) ;
#28229=VERTEX_POINT ( 'NONE', #12691 ) ;
#28231=CIRCLE ( 'NONE', #396, 4.250000000000000000 ) ;
#28262=DIRECTION ( 'NONE',  ( 1.000000000000000000, -0.000000000000000000, -0.000000000000000000 ) ) ;
#28357=VERTEX_POINT ( 'NONE', #6271 ) ;
#28358=AXIS2_PLACEMENT_3D ( 'NONE', #44579, #9462, #25127 ) ;
#28364=EDGE_LOOP ( 'NONE', ( #37945, #46989 ) ) ;
#28395=AXIS2_PLACEMENT_3D ( 'NONE', #22090, #2581, #41090 ) ;
#28408=ORIENTED_EDGE ( 'NONE', *, *, #8052, .T. ) ;
#28428=ADVANCED_FACE ( 'NONE', ( #14711 ), #34227, .T. ) ;
#28463=DIRECTION ( 'NONE',  ( 6.938893903907233900E-15, 0.000000000000000000, -1.000000000000000000 ) ) ;
#28498=CYLINDRICAL_SURFACE ( 'NONE', #13577, 3.750000000000000000 ) ;
#28510=VERTEX_POINT ( 'NONE', #50058 ) ;
#28599=ORIENTED_EDGE ( 'NONE', *, *, #20206, .T. ) ;
#28633=EDGE_CURVE ( 'NONE', #8236, #16307, #20079, .T. ) ;
#28651=ADVANCED_FACE ( 'NONE', ( #43664 ), #43421, .F. ) ;
#28669=VERTEX_POINT ( 'NONE', #5936 ) ;
#28708=ORIENTED_EDGE ( 'NONE', *, *, #15297, .F. ) ;
#28716=( BOUNDED_CURVE ( )  B_SPLINE_CURVE ( 3, ( #48599, #4779, #954, #20691 ),
 .UNSPECIFIED., .F., .F. ) 
 B_SPLINE_CURVE_WITH_KNOTS ( ( 4, 4 ),
 ( 1.570796326794899667, 1.795031077903997518 ),
 .UNSPECIFIED. ) 
 CURVE ( )  GEOMETRIC_REPRESENTATION_ITEM ( )  RATIONAL_B_SPLINE_CURVE ( ( 1.000000000000000000, 0.9958142854328206894, 0.9958142854328206894, 1.000000000000000000 ) ) 
 REPRESENTATION_ITEM ( '' )  );
#28725=EDGE_CURVE ( 'NONE', #16599, #19221, #33655, .T. ) ;
#28742=DIRECTION ( 'NONE',  ( 1.000000000000000000, 0.000000000000000000, 0.000000000000000000 ) ) ;
#28744=ORIENTED_EDGE ( 'NONE', *, *, #23501, .T. ) ;
#28772=CARTESIAN_POINT ( 'NONE',  ( 15.00000000000000000, 8.875661936878623592, 18.94832733001756253 ) ) ;
#28794=CARTESIAN_POINT ( 'NONE',  ( -10.49999999999999467, -46.51315789473684248, -6.315789473684215949 ) ) ;
#28809=DIRECTION ( 'NONE',  ( 0.000000000000000000, 0.000000000000000000, -1.000000000000000000 ) ) ;
#28810=DIRECTION ( 'NONE',  ( -6.938893903907227392E-16, 1.000000000000000000, 0.000000000000000000 ) ) ;
#28824=DIRECTION ( 'NONE',  ( 0.000000000000000000, 0.000000000000000000, 1.000000000000000000 ) ) ;
#28825=FACE_OUTER_BOUND ( 'NONE', #18105, .T. ) ;
#28831=DIRECTION ( 'NONE',  ( 1.000000000000000000, -0.000000000000000000, -0.000000000000000000 ) ) ;
#28837=VECTOR ( 'NONE', #17275, 1000.000000000000000 ) ;
#28849=EDGE_LOOP ( 'NONE', ( #5861, #33580, #46739, #31662 ) ) ;
#28932=AXIS2_PLACEMENT_3D ( 'NONE', #23339, #3840, #23596 ) ;
#28959=EDGE_LOOP ( 'NONE', ( #31367, #15927 ) ) ;
#28963=EDGE_LOOP ( 'NONE', ( #6351, #10459 ) ) ;
#28964=CYLINDRICAL_SURFACE ( 'NONE', #28358, 0.5000000000000004441 ) ;
#29021=ORIENTED_EDGE ( 'NONE', *, *, #3536, .F. ) ;
#29037=ORIENTED_EDGE ( 'NONE', *, *, #9100, .F. ) ;
#29091=DIRECTION ( 'NONE',  ( 6.765175596986472868E-16, -0.9749645535258953943, 0.2223603367690637489 ) ) ;
#29130=CARTESIAN_POINT ( 'NONE',  ( 10.00000000000000178, -46.01315789473684248, 5.916985404131810178 ) ) ;
#29247=AXIS2_PLACEMENT_3D ( 'NONE', #40219, #9419, #9163 ) ;
#29399=ORIENTED_EDGE ( 'NONE', *, *, #38757, .T. ) ;
#29406=ADVANCED_FACE ( 'NONE', ( #25322 ), #13004, .T. ) ;
#29481=EDGE_CURVE ( 'NONE', #24944, #34755, #5053, .T. ) ;
#29493=AXIS2_PLACEMENT_3D ( 'NONE', #36954, #8967, #28222 ) ;
#29511=ORIENTED_EDGE ( 'NONE', *, *, #40037, .F. ) ;
#29513=CYLINDRICAL_SURFACE ( 'NONE', #19609, 0.5000000000000004441 ) ;
#29596=DIRECTION ( 'NONE',  ( -1.000000000000000000, 0.000000000000000000, -0.000000000000000000 ) ) ;
#29621=CARTESIAN_POINT ( 'NONE',  ( -10.01251772323708522, 8.486842105263161073, -18.46084505325461578 ) ) ;
#29623=DIRECTION ( 'NONE',  ( 0.000000000000000000, 0.2223603367690656640, 0.9749645535258950613 ) ) ;
#29638=CARTESIAN_POINT ( 'NONE',  ( 9.999999999999998224, 8.486842105263161073, -18.34680996553532140 ) ) ;
#29652=FACE_OUTER_BOUND ( 'NONE', #9760, .T. ) ;
#29732=DIRECTION ( 'NONE',  ( 1.387778780781444256E-14, -0.000000000000000000, 1.000000000000000000 ) ) ;
#29763=DIRECTION ( 'NONE',  ( 0.000000000000000000, 1.000000000000000000, 8.673617379884027583E-15 ) ) ;
#29786=DIRECTION ( 'NONE',  ( -1.000000000000000000, 0.000000000000000000, 0.000000000000000000 ) ) ;
#29787=AXIS2_PLACEMENT_3D ( 'NONE', #23973, #39628, #20114 ) ;
#29788=ORIENTED_EDGE ( 'NONE', *, *, #1116, .T. ) ;
#29796=AXIS2_PLACEMENT_3D ( 'NONE', #6774, #25775, #49321 ) ;
#29815=CARTESIAN_POINT ( 'NONE',  ( 9.999999999999996447, -34.54492135858216528, 0.000000000000000000 ) ) ;
#29822=ORIENTED_EDGE ( 'NONE', *, *, #15418, .T. ) ;
#29835=VECTOR ( 'NONE', #23833, 1000.000000000000000 ) ;
#29844=DIRECTION ( 'NONE',  ( 0.000000000000000000, 0.000000000000000000, 1.000000000000000000 ) ) ;
#29866=FACE_OUTER_BOUND ( 'NONE', #10180, .T. ) ;
#29884=LINE ( 'NONE', #17826, #4485 ) ;
#29917=ORIENTED_EDGE ( 'NONE', *, *, #44186, .F. ) ;
#29943=CARTESIAN_POINT ( 'NONE',  ( 10.50000000000000178, -46.51315789473684248, 5.916985404131814619 ) ) ;
#29944=AXIS2_PLACEMENT_3D ( 'NONE', #16725, #39091, #8033 ) ;
#29977=DIRECTION ( 'NONE',  ( -6.938893903907227392E-16, 1.000000000000000000, 0.000000000000000000 ) ) ;
#29988=LINE ( 'NONE', #6885, #2654 ) ;
#30067=ADVANCED_FACE ( 'NONE', ( #26148 ), #15371, .T. ) ;
#30102=DIRECTION ( 'NONE',  ( 0.000000000000000000, 1.000000000000000000, 0.000000000000000000 ) ) ;
#30149=DIRECTION ( 'NONE',  ( 0.000000000000000000, -0.000000000000000000, 1.000000000000000000 ) ) ;
#30166=CARTESIAN_POINT ( 'NONE',  ( -15.00199999999999712, -34.54492135858216528, 0.000000000000000000 ) ) ;
#30225=ORIENTED_EDGE ( 'NONE', *, *, #45007, .T. ) ;
#30239=AXIS2_PLACEMENT_3D ( 'NONE', #33845, #13561, #34100 ) ;
#30291=ORIENTED_EDGE ( 'NONE', *, *, #13886, .T. ) ;
#30370=CARTESIAN_POINT ( 'NONE',  ( 15.00000000000000000, -46.01315789473684248, 5.916985404131814619 ) ) ;
#30371=DIRECTION ( 'NONE',  ( 0.000000000000000000, 1.387778780781444256E-14, -1.000000000000000000 ) ) ;
#30381=ORIENTED_EDGE ( 'NONE', *, *, #34364, .F. ) ;
#30407=AXIS2_PLACEMENT_3D ( 'NONE', #24463, #40361, #28809 ) ;
#30456=CIRCLE ( 'NONE', #26357, 5.000000000000000000 ) ;
#30473=AXIS2_PLACEMENT_3D ( 'NONE', #13145, #10057, #37035 ) ;
#30475=DIRECTION ( 'NONE',  ( -1.000000000000000000, -6.938893903907233308E-16, -0.000000000000000000 ) ) ;
#30537=EDGE_CURVE ( 'NONE', #1161, #5556, #27360, .T. ) ;
#30545=ORIENTED_EDGE ( 'NONE', *, *, #39942, .T. ) ;
#30560=VECTOR ( 'NONE', #25894, 1000.000000000000000 ) ;
#30619=VERTEX_POINT ( 'NONE', #36091 ) ;
#30636=VERTEX_POINT ( 'NONE', #32727 ) ;
#30662=DIRECTION ( 'NONE',  ( 0.000000000000000000, 1.000000000000000000, -0.000000000000000000 ) ) ;
#30673=CARTESIAN_POINT ( 'NONE',  ( 10.50000000000000178, -46.51315789473684248, -5.916985404131818171 ) ) ;
#30732=AXIS2_PLACEMENT_3D ( 'NONE', #40393, #5228, #36806 ) ;
#30769=CARTESIAN_POINT ( 'NONE',  ( 15.00000000000000000, -46.51315789473684248, 5.916985404131814619 ) ) ;
#30775=CARTESIAN_POINT ( 'NONE',  ( -10.01251772323708522, 8.486842105263161073, -18.46084505325461578 ) ) ;
#30798=AXIS2_PLACEMENT_3D ( 'NONE', #26781, #31141, #46236 ) ;
#30815=ORIENTED_EDGE ( 'NONE', *, *, #46532, .T. ) ;
#30914=( NAMED_UNIT ( * ) SI_UNIT ( $, .STERADIAN. ) SOLID_ANGLE_UNIT ( ) );
#30919=CARTESIAN_POINT ( 'NONE',  ( 0.000000000000000000, 13.48684210526315930, 0.000000000000000000 ) ) ;
#30993=DIRECTION ( 'NONE',  ( 0.000000000000000000, 0.000000000000000000, -1.000000000000000000 ) ) ;
#31033=PLANE ( 'NONE',  #240 ) ;
#31101=ORIENTED_EDGE ( 'NONE', *, *, #37898, .F. ) ;
#31141=DIRECTION ( 'NONE',  ( -6.765175596986472868E-16, 0.9749645535258953943, 0.2223603367690637489 ) ) ;
#31163=VECTOR ( 'NONE', #28831, 1000.000000000000000 ) ;
#31176=DIRECTION ( 'NONE',  ( 0.000000000000000000, -0.2223603367690656640, -0.9749645535258950613 ) ) ;
#31199=EDGE_LOOP ( 'NONE', ( #29037, #13187, #20686, #35924 ) ) ;
#31213=CARTESIAN_POINT ( 'NONE',  ( -15.00000000000000000, -46.01315789473684248, 6.315789473684215949 ) ) ;
#31247=CARTESIAN_POINT ( 'NONE',  ( 0.000000000000000000, 13.98684210526316107, 0.000000000000000000 ) ) ;
#31266=PLANE ( 'NONE',  #23444 ) ;
#31367=ORIENTED_EDGE ( 'NONE', *, *, #12510, .T. ) ;
#31410=ORIENTED_EDGE ( 'NONE', *, *, #43768, .F. ) ;
#31484=CIRCLE ( 'NONE', #38038, 0.5000000000000004441 ) ;
#31499=DIRECTION ( 'NONE',  ( 1.000000000000000000, 0.000000000000000000, 0.000000000000000000 ) ) ;
#31522=CARTESIAN_POINT ( 'NONE',  ( 9.999999999999998224, 8.486842105263161073, -25.00000000000000000 ) ) ;
#31534=EDGE_CURVE ( 'NONE', #23498, #12400, #430, .T. ) ;
#31554=FACE_OUTER_BOUND ( 'NONE', #5568, .T. ) ;
#31571=ORIENTED_EDGE ( 'NONE', *, *, #43768, .T. ) ;
#31634=CARTESIAN_POINT ( 'NONE',  ( -9.999999999999992895, -48.43825625180578953, 5.363892796379245986 ) ) ;
#31662=ORIENTED_EDGE ( 'NONE', *, *, #49886, .F. ) ;
#31690=VECTOR ( 'NONE', #41344, 1000.000000000000000 ) ;
#31743=CYLINDRICAL_SURFACE ( 'NONE', #316, 0.5000000000000007772 ) ;
#31805=CARTESIAN_POINT ( 'NONE',  ( -14.49999999999999822, 12.98684210526315930, 19.37312575500900280 ) ) ;
#31806=ORIENTED_EDGE ( 'NONE', *, *, #9855, .F. ) ;
#31899=DIRECTION ( 'NONE',  ( 0.000000000000000000, 0.9749645535258953943, 0.2223603367690637489 ) ) ;
#31905=ORIENTED_EDGE ( 'NONE', *, *, #23317, .T. ) ;
#31909=CIRCLE ( 'NONE', #46606, 0.5000000000000004441 ) ;
#31923=CARTESIAN_POINT ( 'NONE',  ( 0.000000000000000000, 0.000000000000000000, 0.000000000000000000 ) ) ;
#31942=EDGE_LOOP ( 'NONE', ( #25140, #6956 ) ) ;
#31952=VERTEX_POINT ( 'NONE', #7052 ) ;
#32078=VECTOR ( 'NONE', #579, 1000.000000000000000 ) ;
#32162=EDGE_CURVE ( 'NONE', #49488, #609, #15435, .T. ) ;
#32174=VECTOR ( 'NONE', #40174, 1000.000000000000000 ) ;
#32181=AXIS2_PLACEMENT_3D ( 'NONE', #19796, #47465, #44144 ) ;
#32188=LINE ( 'NONE', #36304, #48425 ) ;
#32230=CARTESIAN_POINT ( 'NONE',  ( -14.49999999999999822, 12.87566193687862715, 19.86060803177194600 ) ) ;
#32240=CARTESIAN_POINT ( 'NONE',  ( -14.49999999999999822, -46.01315789473684248, -6.315789473684215949 ) ) ;
#32241=CIRCLE ( 'NONE', #21563, 0.5000000000000004441 ) ;
#32330=DIRECTION ( 'NONE',  ( -0.000000000000000000, 1.000000000000000000, -0.000000000000000000 ) ) ;
#32346=VERTEX_POINT ( 'NONE', #11853 ) ;
#32479=ORIENTED_EDGE ( 'NONE', *, *, #36998, .T. ) ;
#32492=LINE ( 'NONE', #9628, #20403 ) ;
#32494=EDGE_CURVE ( 'NONE', #24669, #43275, #47707, .T. ) ;
#32503=AXIS2_PLACEMENT_3D ( 'NONE', #18497, #14135, #6701 ) ;
#32508=CARTESIAN_POINT ( 'NONE',  ( 10.49999999999996447, 8.875661936878630698, 18.94832733001756253 ) ) ;
#32517=ORIENTED_EDGE ( 'NONE', *, *, #3396, .T. ) ;
#32528=EDGE_CURVE ( 'NONE', #30619, #27759, #35163, .T. ) ;
#32649=CARTESIAN_POINT ( 'NONE',  ( 10.01251772323701594, 8.486842105263161073, -18.46084505325461578 ) ) ;
#32676=CARTESIAN_POINT ( 'NONE',  ( -14.49999999999999822, 12.98684210526315930, 19.37312575500899925 ) ) ;
#32682=EDGE_CURVE ( 'NONE', #576, #13837, #37989, .T. ) ;
#32709=EDGE_LOOP ( 'NONE', ( #45785, #39225, #27270 ) ) ;
#32723=CARTESIAN_POINT ( 'NONE',  ( 14.49999999999999822, -46.51315789473684248, 5.916985404131814619 ) ) ;
#32727=CARTESIAN_POINT ( 'NONE',  ( 6.123233995736766282E-16, 28.48684210526315752, 5.000000000000000000 ) ) ;
#32786=ORIENTED_EDGE ( 'NONE', *, *, #1116, .F. ) ;
#32805=CARTESIAN_POINT ( 'NONE',  ( 0.000000000000000000, 23.48684210526316107, 0.000000000000000000 ) ) ;
#32840=FACE_OUTER_BOUND ( 'NONE', #35316, .T. ) ;
#32845=AXIS2_PLACEMENT_3D ( 'NONE', #35232, #39332, #75 ) ;
#32869=DIRECTION ( 'NONE',  ( 0.000000000000000000, -1.000000000000000000, 0.000000000000000000 ) ) ;
#32881=LINE ( 'NONE', #36225, #23352 ) ;
#32897=EDGE_LOOP ( 'NONE', ( #22716, #8358, #13593, #47730 ) ) ;
#32923=CARTESIAN_POINT ( 'NONE',  ( -14.49999999999999822, 12.98684210526315930, 19.37312575500900280 ) ) ;
#32978=SPHERICAL_SURFACE ( 'NONE', #2930, 0.5000000000000000000 ) ;
#32994=LINE ( 'NONE', #16825, #17234 ) ;
#33011=CARTESIAN_POINT ( 'NONE',  ( -14.49999999999999822, 13.48684210526315930, -19.37312575500899570 ) ) ;
#33027=ORIENTED_EDGE ( 'NONE', *, *, #3855, .F. ) ;
#33028=ORIENTED_EDGE ( 'NONE', *, *, #38493, .F. ) ;
#33064=EDGE_CURVE ( 'NONE', #1662, #576, #7828, .T. ) ;
#33078=( BOUNDED_CURVE ( )  B_SPLINE_CURVE ( 3, ( #35062, #22717, #38388, #3200 ),
 .UNSPECIFIED., .F., .F. ) 
 B_SPLINE_CURVE_WITH_KNOTS ( ( 4, 4 ),
 ( 1.570796326794891673, 2.917357902480690601 ),
 .UNSPECIFIED. ) 
 CURVE ( )  GEOMETRIC_REPRESENTATION_ITEM ( )  RATIONAL_B_SPLINE_CURVE ( ( 1.000000000000000000, 0.8545200852688804583, 0.8545200852688804583, 1.000000000000000000 ) ) 
 REPRESENTATION_ITEM ( '' )  );
#33107=ORIENTED_EDGE ( 'NONE', *, *, #9855, .T. ) ;
#33110=CARTESIAN_POINT ( 'NONE',  ( 14.49999999999999822, 12.98684210526315930, 19.37312575500900280 ) ) ;
#33190=VECTOR ( 'NONE', #49274, 1000.000000000000000 ) ;
#33233=LINE ( 'NONE', #48815, #41442 ) ;
#33309=SPHERICAL_SURFACE ( 'NONE', #23262, 0.5000000000000000000 ) ;
#33362=EDGE_CURVE ( 'NONE', #18141, #24669, #23409, .T. ) ;
#33501=ADVANCED_FACE ( 'NONE', ( #17085 ), #13228, .T. ) ;
#33580=ORIENTED_EDGE ( 'NONE', *, *, #38861, .T. ) ;
#33581=ADVANCED_FACE ( 'NONE', ( #14750, #2932 ), #37619, .F. ) ;
#33634=CARTESIAN_POINT ( 'NONE',  ( -14.49999999999999822, 12.98684210526315930, 19.37312575500900280 ) ) ;
#33655=LINE ( 'NONE', #28794, #31690 ) ;
#33659=CARTESIAN_POINT ( 'NONE',  ( -10.50000000000003375, 8.875661936878628921, -18.94832733001756253 ) ) ;
#33666=DIRECTION ( 'NONE',  ( 0.000000000000000000, 0.9749645535258947282, 0.2223603367690671906 ) ) ;
#33677=EDGE_CURVE ( 'NONE', #34075, #38020, #2494, .T. ) ;
#33679=VECTOR ( 'NONE', #5605, 1000.000000000000000 ) ;
#33702=EDGE_CURVE ( 'NONE', #30636, #46117, #18020, .T. ) ;
#33750=ORIENTED_EDGE ( 'NONE', *, *, #32528, .T. ) ;
#33751=ADVANCED_FACE ( 'NONE', ( #20367 ), #19859, .T. ) ;
#33759=EDGE_CURVE ( 'NONE', #19764, #28669, #20118, .T. ) ;
#33761=CARTESIAN_POINT ( 'NONE',  ( 10.01251772323701594, 8.486842105263161073, -18.46084505325461578 ) ) ;
#33775=ADVANCED_FACE ( 'NONE', ( #633 ), #23477, .T. ) ;
#33824=EDGE_CURVE ( 'NONE', #42504, #16599, #13680, .T. ) ;
#33845=CARTESIAN_POINT ( 'NONE',  ( 0.000000000000000000, 28.48684210526315752, 0.000000000000000000 ) ) ;
#33850=LINE ( 'NONE', #10233, #30560 ) ;
#33954=CARTESIAN_POINT ( 'NONE',  ( -14.49999999999999822, 13.48684210526315930, 19.37312575500900280 ) ) ;
#34036=ORIENTED_EDGE ( 'NONE', *, *, #15258, .T. ) ;
#34070=ADVANCED_FACE ( 'NONE', ( #14685 ), #2383, .T. ) ;
#34074=AXIS2_PLACEMENT_3D ( 'NONE', #33110, #40290, #28742 ) ;
#34075=VERTEX_POINT ( 'NONE', #34458 ) ;
#34082=EDGE_CURVE ( 'NONE', #46117, #39523, #18026, .T. ) ;
#34100=DIRECTION ( 'NONE',  ( 0.000000000000000000, 0.000000000000000000, -1.000000000000000000 ) ) ;
#34112=ORIENTED_EDGE ( 'NONE', *, *, #15418, .F. ) ;
#34158=CARTESIAN_POINT ( 'NONE',  ( -14.49999999999999822, -46.01315789473684248, -5.916985404131814619 ) ) ;
#34222=DIRECTION ( 'NONE',  ( 0.000000000000000000, 0.9749645535258953943, -0.2223603367690637489 ) ) ;
#34227=CYLINDRICAL_SURFACE ( 'NONE', #10353, 0.5000000000000004441 ) ;
#34232=CYLINDRICAL_SURFACE ( 'NONE', #30798, 0.4999999999999997224 ) ;
#34273=DIRECTION ( 'NONE',  ( 0.000000000000000000, 0.000000000000000000, -1.000000000000000000 ) ) ;
#34327=CARTESIAN_POINT ( 'NONE',  ( 9.999999999999996447, -34.54492135858216528, 0.000000000000000000 ) ) ;
#34364=EDGE_CURVE ( 'NONE', #18141, #46782, #9859, .T. ) ;
#34381=AXIS2_PLACEMENT_3D ( 'NONE', #47620, #28173, #8678 ) ;
#34403=EDGE_LOOP ( 'NONE', ( #9016, #14129, #25192, #460, #42728 ) ) ;
#34407=PLANE ( 'NONE',  #18504 ) ;
#34458=CARTESIAN_POINT ( 'NONE',  ( 10.01251772323701594, 8.486842105263161073, -18.46084505325461578 ) ) ;
#34468=CARTESIAN_POINT ( 'NONE',  ( -9.999999999999998224, 8.486842105263161073, -25.00000000000000000 ) ) ;
#34625=DIRECTION ( 'NONE',  ( 0.000000000000000000, -0.000000000000000000, 1.000000000000000000 ) ) ;
#34740=EDGE_LOOP ( 'NONE', ( #45839, #33750, #33027 ) ) ;
#34755=VERTEX_POINT ( 'NONE', #25360 ) ;
#34846=LINE ( 'NONE', #50427, #1634 ) ;
#34851=CYLINDRICAL_SURFACE ( 'NONE', #43675, 0.5000000000000004441 ) ;
#34883=DIRECTION ( 'NONE',  ( 0.000000000000000000, 1.000000000000000000, -0.000000000000000000 ) ) ;
#34886=CIRCLE ( 'NONE', #12738, 4.999999999999997335 ) ;
#34948=LINE ( 'NONE', #2842, #19725 ) ;
#34961=VECTOR ( 'NONE', #3209, 1000.000000000000000 ) ;
#35026=DIRECTION ( 'NONE',  ( 1.000000000000000000, 0.000000000000000000, 0.000000000000000000 ) ) ;
#35042=CARTESIAN_POINT ( 'NONE',  ( 10.00000000000000178, -46.01315789473684248, -25.00000000000000000 ) ) ;
#35062=CARTESIAN_POINT ( 'NONE',  ( -10.50000000000003375, 8.875661936878630698, 18.94832733001756253 ) ) ;
#35072=CARTESIAN_POINT ( 'NONE',  ( 15.00000000000000000, -46.51315789473684248, -5.916985404131818171 ) ) ;
#35093=FACE_OUTER_BOUND ( 'NONE', #24893, .T. ) ;
#35162=DIRECTION ( 'NONE',  ( 0.000000000000000000, 1.000000000000000000, 0.000000000000000000 ) ) ;
#35163=CIRCLE ( 'NONE', #24526, 0.5000000000000004441 ) ;
#35204=DIRECTION ( 'NONE',  ( 0.000000000000000000, -0.9749645535258953943, -0.2223603367690637489 ) ) ;
#35213=ORIENTED_EDGE ( 'NONE', *, *, #7740, .T. ) ;
#35232=CARTESIAN_POINT ( 'NONE',  ( -14.49999999999999822, 12.98684210526315930, -19.37312575500899570 ) ) ;
#35236=SPHERICAL_SURFACE ( 'NONE', #29944, 0.5000000000000000000 ) ;
#35239=ORIENTED_EDGE ( 'NONE', *, *, #36343, .T. ) ;
#35245=DIRECTION ( 'NONE',  ( 0.000000000000000000, 0.000000000000000000, 1.000000000000000000 ) ) ;
#35275=SHAPE_REPRESENTATION ( 'tire holder', ( #45486 ), #13533 ) ;
#35305=CIRCLE ( 'NONE', #32845, 0.5000000000000004441 ) ;
#35316=EDGE_LOOP ( 'NONE', ( #7412, #48467, #30545, #31806 ) ) ;
#35368=ORIENTED_EDGE ( 'NONE', *, *, #46516, .T. ) ;
#35396=DIRECTION ( 'NONE',  ( -1.000000000000000000, 0.000000000000000000, 0.000000000000000000 ) ) ;
#35407=DIRECTION ( 'NONE',  ( -0.000000000000000000, 1.000000000000000000, 0.000000000000000000 ) ) ;
#35437=ORIENTED_EDGE ( 'NONE', *, *, #50333, .F. ) ;
#35530=EDGE_LOOP ( 'NONE', ( #9103, #36576, #46393, #4996 ) ) ;
#35582=ORIENTED_EDGE ( 'NONE', *, *, #8880, .F. ) ;
#35622=DIRECTION ( 'NONE',  ( -0.000000000000000000, 0.9749645535258956164, 0.2223603367690631105 ) ) ;
#35635=ADVANCED_FACE ( 'NONE', ( #50498 ), #15652, .T. ) ;
#35640=VERTEX_POINT ( 'NONE', #23348 ) ;
#35650=ADVANCED_FACE ( 'NONE', ( #12814 ), #9211, .T. ) ;
#35672=CARTESIAN_POINT ( 'NONE',  ( -10.49999999999999467, -46.51315789473684248, 5.916985404131814619 ) ) ;
#35683=CYLINDRICAL_SURFACE ( 'NONE', #10145, 0.5000000000000004441 ) ;
#35693=DIRECTION ( 'NONE',  ( 0.000000000000000000, 0.000000000000000000, 1.000000000000000000 ) ) ;
#35772=ADVANCED_FACE ( 'NONE', ( #13305 ), #28964, .T. ) ;
#35851=CARTESIAN_POINT ( 'NONE',  ( 14.49999999999999822, -3.557843729863133575, 15.59977635401528673 ) ) ;
#35854=CYLINDRICAL_SURFACE ( 'NONE', #14027, 0.5000000000000004441 ) ;
#35857=DIRECTION ( 'NONE',  ( 0.000000000000000000, 0.9749645535258955054, 0.2223603367690637767 ) ) ;
#35881=VERTEX_POINT ( 'NONE', #2025 ) ;
#35924=ORIENTED_EDGE ( 'NONE', *, *, #36998, .F. ) ;
#35926=VERTEX_POINT ( 'NONE', #46850 ) ;
#35957=FACE_OUTER_BOUND ( 'NONE', #24767, .T. ) ;
#36011=AXIS2_PLACEMENT_3D ( 'NONE', #41620, #10820, #26472 ) ;
#36012=VECTOR ( 'NONE', #37705, 1000.000000000000000 ) ;
#36041=EDGE_CURVE ( 'NONE', #37345, #28357, #9854, .T. ) ;
#36091=CARTESIAN_POINT ( 'NONE',  ( -14.49999999999999822, -46.51315789473684248, 5.916985404131814619 ) ) ;
#36162=SPHERICAL_SURFACE ( 'NONE', #8407, 0.5000000000000000000 ) ;
#36225=CARTESIAN_POINT ( 'NONE',  ( 14.49999999999999822, -46.51315789473684248, 6.315789473684215949 ) ) ;
#36304=CARTESIAN_POINT ( 'NONE',  ( 4.592425496802573972E-16, 23.48684210526316107, 3.750000000000000000 ) ) ;
#36319=CYLINDRICAL_SURFACE ( 'NONE', #37105, 0.4999999999999992228 ) ;
#36343=EDGE_CURVE ( 'NONE', #3066, #20304, #33078, .T. ) ;
#36398=CIRCLE ( 'NONE', #24081, 0.4999999999999997224 ) ;
#36441=ORIENTED_EDGE ( 'NONE', *, *, #24735, .F. ) ;
#36463=AXIS2_PLACEMENT_3D ( 'NONE', #18673, #18170, #14836 ) ;
#36478=ADVANCED_FACE ( 'NONE', ( #20644 ), #36319, .T. ) ;
#36532=VECTOR ( 'NONE', #40060, 1000.000000000000000 ) ;
#36576=ORIENTED_EDGE ( 'NONE', *, *, #15297, .T. ) ;
#36604=ORIENTED_EDGE ( 'NONE', *, *, #37898, .T. ) ;
#36662=CARTESIAN_POINT ( 'NONE',  ( 0.000000000000000000, 28.48684210526315752, 0.000000000000000000 ) ) ;
#36718=DIRECTION ( 'NONE',  ( 0.000000000000000000, 0.9749645535258959494, 0.2223603367690620558 ) ) ;
#36733=DIRECTION ( 'NONE',  ( 0.000000000000000000, 0.000000000000000000, -1.000000000000000000 ) ) ;
#36748=VECTOR ( 'NONE', #15056, 1000.000000000000000 ) ;
#36779=ORIENTED_EDGE ( 'NONE', *, *, #37829, .T. ) ;
#36797=CARTESIAN_POINT ( 'NONE',  ( -10.00000000000000178, -37.59858392880988731, -7.836098764781820769 ) ) ;
#36806=DIRECTION ( 'NONE',  ( 0.000000000000000000, 0.2223603367690619725, -0.9749645535258958384 ) ) ;
#36890=ADVANCED_FACE ( 'NONE', ( #48676 ), #44352, .T. ) ;
#36920=EDGE_CURVE ( 'NONE', #28510, #16010, #21540, .T. ) ;
#36954=CARTESIAN_POINT ( 'NONE',  ( -14.49999999999999822, 12.98684210526315930, 19.37312575500900280 ) ) ;
#36987=SHAPE_DEFINITION_REPRESENTATION ( #9731, #35275 ) ;
#36998=EDGE_CURVE ( 'NONE', #5426, #7866, #33850, .T. ) ;
#37035=DIRECTION ( 'NONE',  ( 0.000000000000000000, -0.9749645535258953943, 0.2223603367690637489 ) ) ;
#37062=VECTOR ( 'NONE', #22043, 1000.000000000000000 ) ;
#37105=AXIS2_PLACEMENT_3D ( 'NONE', #20896, #44473, #23996 ) ;
#37345=VERTEX_POINT ( 'NONE', #14428 ) ;
#37346=AXIS2_PLACEMENT_3D ( 'NONE', #27746, #7746, #4395 ) ;
#37431=DIRECTION ( 'NONE',  ( 1.000000000000000000, 0.000000000000000000, -1.224646799147353207E-16 ) ) ;
#37496=DIRECTION ( 'NONE',  ( 0.000000000000000000, 0.000000000000000000, 1.000000000000000000 ) ) ;
#37619=PLANE ( 'NONE',  #48277 ) ;
#37633=DIRECTION ( 'NONE',  ( -0.000000000000000000, 1.000000000000000000, 0.000000000000000000 ) ) ;
#37643=AXIS2_PLACEMENT_3D ( 'NONE', #5662, #4900, #9512 ) ;
#37653=AXIS2_PLACEMENT_3D ( 'NONE', #25142, #36718, #45104 ) ;
#37685=ORIENTED_EDGE ( 'NONE', *, *, #7417, .F. ) ;
#37697=VERTEX_POINT ( 'NONE', #45634 ) ;
#37705=DIRECTION ( 'NONE',  ( 1.000000000000000000, -0.000000000000000000, -0.000000000000000000 ) ) ;
#37750=EDGE_CURVE ( 'NONE', #11655, #1161, #50199, .T. ) ;
#37829=EDGE_CURVE ( 'NONE', #49488, #35926, #45281, .T. ) ;
#37838=ORIENTED_EDGE ( 'NONE', *, *, #47195, .T. ) ;
#37840=CIRCLE ( 'NONE', #1780, 0.5000000000000004441 ) ;
#37842=FACE_OUTER_BOUND ( 'NONE', #42274, .T. ) ;
#37879=DIRECTION ( 'NONE',  ( 0.000000000000000000, 0.000000000000000000, -1.000000000000000000 ) ) ;
#37898=EDGE_CURVE ( 'NONE', #9479, #47807, #42847, .T. ) ;
#37945=ORIENTED_EDGE ( 'NONE', *, *, #21525, .F. ) ;
#37989=LINE ( 'NONE', #3830, #44132 ) ;
#37993=EDGE_LOOP ( 'NONE', ( #42382, #10386 ) ) ;
#38020=VERTEX_POINT ( 'NONE', #29638 ) ;
#38038=AXIS2_PLACEMENT_3D ( 'NONE', #12982, #9651, #17348 ) ;
#38080=CARTESIAN_POINT ( 'NONE',  ( -14.49999999999999822, 12.98684210526315930, -19.37312575500900280 ) ) ;
#38109=ADVANCED_FACE ( 'NONE', ( #11923 ), #38367, .T. ) ;
#38163=EDGE_LOOP ( 'NONE', ( #34036, #37685, #32786, #29511, #39543 ) ) ;
#38181=ADVANCED_FACE ( 'NONE', ( #47280 ), #27825, .F. ) ;
#38183=CIRCLE ( 'NONE', #22589, 5.000000000000000888 ) ;
#38318=DIRECTION ( 'NONE',  ( 0.000000000000000000, 0.000000000000000000, 1.000000000000000000 ) ) ;
#38359=DIRECTION ( 'NONE',  ( -6.765175596986471882E-16, 0.9749645535258953943, 0.2223603367690637489 ) ) ;
#38361=FACE_OUTER_BOUND ( 'NONE', #3786, .T. ) ;
#38367=SPHERICAL_SURFACE ( 'NONE', #26405, 0.5000000000000000000 ) ;
#38369=EDGE_CURVE ( 'NONE', #37697, #40121, #39073, .T. ) ;
#38388=CARTESIAN_POINT ( 'NONE',  ( -10.06660411345808548, 8.486842105263157521, 18.70408263333243681 ) ) ;
#38398=LINE ( 'NONE', #3990, #34961 ) ;
#38408=EDGE_CURVE ( 'NONE', #28669, #576, #1843, .T. ) ;
#38489=DIRECTION ( 'NONE',  ( 0.000000000000000000, 1.000000000000000000, 0.000000000000000000 ) ) ;
#38493=EDGE_CURVE ( 'NONE', #8236, #35926, #10043, .T. ) ;
#38563=AXIS2_PLACEMENT_3D ( 'NONE', #34158, #17958, #49729 ) ;
#38612=( LENGTH_UNIT ( ) NAMED_UNIT ( * ) SI_UNIT ( .MILLI., .METRE. ) );
#38667=ORIENTED_EDGE ( 'NONE', *, *, #42744, .F. ) ;
#38750=ADVANCED_FACE ( 'NONE', ( #751 ), #36162, .T. ) ;
#38755=FACE_BOUND ( 'NONE', #27855, .T. ) ;
#38757=EDGE_CURVE ( 'NONE', #30619, #42504, #261, .T. ) ;
#38758=ORIENTED_EDGE ( 'NONE', *, *, #17761, .F. ) ;
#38854=ORIENTED_EDGE ( 'NONE', *, *, #33362, .F. ) ;
#38861=EDGE_CURVE ( 'NONE', #47807, #31952, #17473, .T. ) ;
#38867=AXIS2_PLACEMENT_3D ( 'NONE', #990, #9935, #24586 ) ;
#38879=AXIS2_PLACEMENT_3D ( 'NONE', #43857, #43108, #35693 ) ;
#38883=VECTOR ( 'NONE', #21319, 1000.000000000000000 ) ;
#38902=CARTESIAN_POINT ( 'NONE',  ( -14.49999999999999822, 12.98684210526315930, 19.37312575500899925 ) ) ;
#38905=ORIENTED_EDGE ( 'NONE', *, *, #1792, .F. ) ;
#38908=DIRECTION ( 'NONE',  ( 1.000000000000000000, 6.938893903907233308E-16, 0.000000000000000000 ) ) ;
#38917=LINE ( 'NONE', #31213, #22432 ) ;
#38940=FACE_OUTER_BOUND ( 'NONE', #14570, .T. ) ;
#38986=CARTESIAN_POINT ( 'NONE',  ( 14.49999999999999822, 13.48684210526315930, 20.00000000000000000 ) ) ;
#39028=DIRECTION ( 'NONE',  ( 1.000000000000000000, 0.000000000000000000, 0.000000000000000000 ) ) ;
#39057=DIRECTION ( 'NONE',  ( -0.000000000000000000, -0.000000000000000000, 1.000000000000000000 ) ) ;
#39073=LINE ( 'NONE', #42630, #45200 ) ;
#39091=DIRECTION ( 'NONE',  ( 0.000000000000000000, 1.000000000000000000, -0.000000000000000000 ) ) ;
#39173=VERTEX_POINT ( 'NONE', #33011 ) ;
#39200=CARTESIAN_POINT ( 'NONE',  ( 14.49999999999999822, -46.01315789473684248, -5.916985404131818171 ) ) ;
#39202=ORIENTED_EDGE ( 'NONE', *, *, #38369, .T. ) ;
#39225=ORIENTED_EDGE ( 'NONE', *, *, #47742, .T. ) ;
#39230=CLOSED_SHELL ( 'NONE', ( #45207, #25344, #50075, #20269, #1561, #33775, #28003, #45243, #28651, #38181, #43760, #47291, #45082, #2605, #26003, #27698, #22686, #23531, #21725, #8972, #14599, #33581, #33751, #20443, #34070, #46481, #35772, #25296, #33501, #12963, #36478, #47811, #43551, #8051, #2075, #41302, #27415, #38750, #30067, #13430, #10259, #39702, #28428, #6426, #17833, #38109, #14185, #46478, #35650, #36890, #42606, #45784, #35635, #26814, #9882, #29406, #18607 ) ) ;
#39245=DIRECTION ( 'NONE',  ( 0.000000000000000000, -0.2223603367690619725, -0.9749645535258958384 ) ) ;
#39332=DIRECTION ( 'NONE',  ( 1.000000000000000000, -0.000000000000000000, 0.000000000000000000 ) ) ;
#39343=CIRCLE ( 'NONE', #17208, 3.750000000000000000 ) ;
#39523=VERTEX_POINT ( 'NONE', #15647 ) ;
#39543=ORIENTED_EDGE ( 'NONE', *, *, #32494, .F. ) ;
#39628=DIRECTION ( 'NONE',  ( 0.000000000000000000, 1.000000000000000000, 0.000000000000000000 ) ) ;
#39631=DIRECTION ( 'NONE',  ( 6.765175596986472868E-16, -0.9749645535258953943, 0.2223603367690637489 ) ) ;
#39639=DIRECTION ( 'NONE',  ( -6.765175596986471882E-16, 0.9749645535258953943, -0.2223603367690637489 ) ) ;
#39648=AXIS2_PLACEMENT_3D ( 'NONE', #32805, #24098, #16636 ) ;
#39702=ADVANCED_FACE ( 'NONE', ( #4104 ), #35683, .T. ) ;
#39753=SPHERICAL_SURFACE ( 'NONE', #7703, 0.5000000000000000000 ) ;
#39762=ORIENTED_EDGE ( 'NONE', *, *, #7417, .T. ) ;
#39795=ORIENTED_EDGE ( 'NONE', *, *, #47742, .F. ) ;
#39806=PLANE ( 'NONE',  #25647 ) ;
#39808=ORIENTED_EDGE ( 'NONE', *, *, #9182, .F. ) ;
#39813=CARTESIAN_POINT ( 'NONE',  ( -15.00199999999999712, -34.54492135858216528, 5.000000000000000000 ) ) ;
#39865=CIRCLE ( 'NONE', #19365, 4.999999999999997335 ) ;
#39942=EDGE_CURVE ( 'NONE', #6443, #16093, #47797, .T. ) ;
#39960=EDGE_CURVE ( 'NONE', #28669, #37345, #4544, .T. ) ;
#39966=( BOUNDED_CURVE ( )  B_SPLINE_CURVE ( 3, ( #32649, #41096, #5940, #21588 ),
 .UNSPECIFIED., .F., .F. ) 
 B_SPLINE_CURVE_WITH_KNOTS ( ( 4, 4 ),
 ( 0.2242347511090889423, 1.570796326794895670 ),
 .UNSPECIFIED. ) 
 CURVE ( )  GEOMETRIC_REPRESENTATION_ITEM ( )  RATIONAL_B_SPLINE_CURVE ( ( 1.000000000000000000, 0.8545200852688790150, 0.8545200852688790150, 1.000000000000000000 ) ) 
 REPRESENTATION_ITEM ( '' )  );
#40015=EDGE_CURVE ( 'NONE', #26840, #16599, #21609, .T. ) ;
#40037=EDGE_CURVE ( 'NONE', #43275, #10525, #31484, .T. ) ;
#40060=DIRECTION ( 'NONE',  ( 1.000000000000000000, -0.000000000000000000, -0.000000000000000000 ) ) ;
#40121=VERTEX_POINT ( 'NONE', #27095 ) ;
#40158=EDGE_LOOP ( 'NONE', ( #44533, #22962, #46603 ) ) ;
#40174=DIRECTION ( 'NONE',  ( -1.000000000000000000, 0.000000000000000000, 0.000000000000000000 ) ) ;
#40194=PLANE ( 'NONE',  #40994 ) ;
#40201=DIRECTION ( 'NONE',  ( 1.000000000000000000, -0.000000000000000000, -0.000000000000000000 ) ) ;
#40219=CARTESIAN_POINT ( 'NONE',  ( 14.49999999999999822, 12.98684210526315930, 0.000000000000000000 ) ) ;
#40290=DIRECTION ( 'NONE',  ( -0.000000000000000000, -0.000000000000000000, -1.000000000000000000 ) ) ;
#40318=EDGE_LOOP ( 'NONE', ( #25468, #2510, #6731, #2478 ) ) ;
#40357=ORIENTED_EDGE ( 'NONE', *, *, #10641, .T. ) ;
#40361=DIRECTION ( 'NONE',  ( 1.000000000000000000, 0.000000000000000000, -0.000000000000000000 ) ) ;
#40393=CARTESIAN_POINT ( 'NONE',  ( -10.49999999999999467, -46.01315789473684248, 5.916985404131813731 ) ) ;
#40464=CIRCLE ( 'NONE', #29796, 0.5000000000000004441 ) ;
#40640=ORIENTED_EDGE ( 'NONE', *, *, #49886, .T. ) ;
#40643=CARTESIAN_POINT ( 'NONE',  ( 9.999999999999994671, -37.59858392880989442, -7.836098764781824322 ) ) ;
#40686=DIRECTION ( 'NONE',  ( -0.000000000000000000, 0.9749645535258953943, 0.2223603367690637489 ) ) ;
#40994=AXIS2_PLACEMENT_3D ( 'NONE', #20945, #47339, #12231 ) ;
#41090=DIRECTION ( 'NONE',  ( 0.000000000000000000, 0.000000000000000000, 1.000000000000000000 ) ) ;
#41096=CARTESIAN_POINT ( 'NONE',  ( 10.06660411345801087, 8.486842105263159297, -18.70408263333243326 ) ) ;
#41161=ORIENTED_EDGE ( 'NONE', *, *, #25079, .F. ) ;
#41183=CIRCLE ( 'NONE', #7618, 0.4999999999999995559 ) ;
#41193=SPHERICAL_SURFACE ( 'NONE', #6977, 0.5000000000000000000 ) ;
#41196=CARTESIAN_POINT ( 'NONE',  ( -10.49999999999999467, -46.01315789473684248, -5.916985404131814619 ) ) ;
#41202=AXIS2_PLACEMENT_3D ( 'NONE', #16666, #24880, #44102 ) ;
#41302=ADVANCED_FACE ( 'NONE', ( #21164 ), #1182, .T. ) ;
#41344=DIRECTION ( 'NONE',  ( 0.000000000000000000, -0.000000000000000000, 1.000000000000000000 ) ) ;
#41376=AXIS2_PLACEMENT_3D ( 'NONE', #17526, #4964, #21368 ) ;
#41386=DIRECTION ( 'NONE',  ( 1.000000000000000000, 0.000000000000000000, 0.000000000000000000 ) ) ;
#41442=VECTOR ( 'NONE', #13455, 1000.000000000000114 ) ;
#41470=DIRECTION ( 'NONE',  ( -1.000000000000000000, 0.000000000000000000, 0.000000000000000000 ) ) ;
#41483=DIRECTION ( 'NONE',  ( 6.938893903907232322E-16, -1.000000000000000000, 0.000000000000000000 ) ) ;
#41484=ORIENTED_EDGE ( 'NONE', *, *, #47440, .F. ) ;
#41494=EDGE_CURVE ( 'NONE', #28510, #43275, #50383, .T. ) ;
#41545=ORIENTED_EDGE ( 'NONE', *, *, #4687, .T. ) ;
#41602=FACE_OUTER_BOUND ( 'NONE', #12415, .T. ) ;
#41620=CARTESIAN_POINT ( 'NONE',  ( 14.49999999999999822, 12.98684210526315930, -19.37312575500900280 ) ) ;
#41734=CARTESIAN_POINT ( 'NONE',  ( -10.00000000000000355, -34.54492135858216528, 0.000000000000000000 ) ) ;
#41875=DIRECTION ( 'NONE',  ( 0.000000000000000000, 0.000000000000000000, 1.000000000000000000 ) ) ;
#41903=ORIENTED_EDGE ( 'NONE', *, *, #8504, .F. ) ;
#41917=CARTESIAN_POINT ( 'NONE',  ( -10.01251772323708700, 8.486842105263161073, 18.46084505325461578 ) ) ;
#41986=DIRECTION ( 'NONE',  ( 1.000000000000000000, 6.938893903907233308E-16, 0.000000000000000000 ) ) ;
#42050=AXIS2_PLACEMENT_3D ( 'NONE', #42317, #19208, #29763 ) ;
#42064=DIRECTION ( 'NONE',  ( -6.765175596986472868E-16, 0.9749645535258953943, 0.2223603367690637489 ) ) ;
#42107=AXIS2_PLACEMENT_3D ( 'NONE', #34327, #30475, #29977 ) ;
#42115=CARTESIAN_POINT ( 'NONE',  ( -14.49999999999999822, 13.48684210526315930, 20.00000000000000000 ) ) ;
#42127=CARTESIAN_POINT ( 'NONE',  ( -10.49999999999999467, -46.01315789473684248, -6.315789473684215949 ) ) ;
#42182=VERTEX_POINT ( 'NONE', #50145 ) ;
#42274=EDGE_LOOP ( 'NONE', ( #44459, #34112, #10404, #42649, #35437 ) ) ;
#42317=CARTESIAN_POINT ( 'NONE',  ( 14.49999999999999822, -46.01315789473684248, -5.916985404131813731 ) ) ;
#42335=EDGE_LOOP ( 'NONE', ( #18206, #48792, #12397, #49152 ) ) ;
#42340=FACE_BOUND ( 'NONE', #37993, .T. ) ;
#42382=ORIENTED_EDGE ( 'NONE', *, *, #24326, .F. ) ;
#42454=VERTEX_POINT ( 'NONE', #21419 ) ;
#42504=VERTEX_POINT ( 'NONE', #7820 ) ;
#42606=ADVANCED_FACE ( 'NONE', ( #38361 ), #3173, .T. ) ;
#42630=CARTESIAN_POINT ( 'NONE',  ( 15.00000000000000000, -46.12433806312137108, -6.404467680894764925 ) ) ;
#42649=ORIENTED_EDGE ( 'NONE', *, *, #25817, .F. ) ;
#42684=ORIENTED_EDGE ( 'NONE', *, *, #16150, .T. ) ;
#42728=ORIENTED_EDGE ( 'NONE', *, *, #33677, .F. ) ;
#42740=DIRECTION ( 'NONE',  ( 0.000000000000000000, 0.2223603367690632493, -0.9749645535258955054 ) ) ;
#42744=EDGE_CURVE ( 'NONE', #26840, #12918, #47770, .T. ) ;
#42765=CARTESIAN_POINT ( 'NONE',  ( 14.49999999999999822, -46.01315789473684248, 5.916985404131814619 ) ) ;
#42838=AXIS2_PLACEMENT_3D ( 'NONE', #17202, #32869, #36733 ) ;
#42842=CARTESIAN_POINT ( 'NONE',  ( 14.49999999999999822, -46.01315789473684248, 5.916985404131813731 ) ) ;
#42847=CIRCLE ( 'NONE', #5167, 4.250000000000000000 ) ;
#43027=DIRECTION ( 'NONE',  ( 1.000000000000000000, 0.000000000000000000, 3.469446951953611033E-15 ) ) ;
#43041=ORIENTED_EDGE ( 'NONE', *, *, #25208, .F. ) ;
#43069=AXIS2_PLACEMENT_3D ( 'NONE', #18596, #37633, #34273 ) ;
#43084=DIRECTION ( 'NONE',  ( -6.938893903907233900E-15, 0.000000000000000000, 1.000000000000000000 ) ) ;
#43108=DIRECTION ( 'NONE',  ( -1.000000000000000000, 0.000000000000000000, 0.000000000000000000 ) ) ;
#43255=DIRECTION ( 'NONE',  ( -0.000000000000000000, -0.000000000000000000, 1.000000000000000000 ) ) ;
#43272=CYLINDRICAL_SURFACE ( 'NONE', #2540, 0.4999999999999997224 ) ;
#43275=VERTEX_POINT ( 'NONE', #21554 ) ;
#43421=PLANE ( 'NONE',  #21006 ) ;
#43436=CARTESIAN_POINT ( 'NONE',  ( -15.00000000000000000, -46.40197772635230677, -5.828307196921269195 ) ) ;
#43437=VERTEX_POINT ( 'NONE', #49630 ) ;
#43481=ORIENTED_EDGE ( 'NONE', *, *, #20236, .T. ) ;
#43515=FACE_OUTER_BOUND ( 'NONE', #819, .T. ) ;
#43526=DIRECTION ( 'NONE',  ( -0.000000000000000000, 1.000000000000000000, -0.000000000000000000 ) ) ;
#43527=DIRECTION ( 'NONE',  ( 0.000000000000000000, 0.000000000000000000, -1.000000000000000000 ) ) ;
#43551=ADVANCED_FACE ( 'NONE', ( #7275 ), #22921, .T. ) ;
#43650=AXIS2_PLACEMENT_3D ( 'NONE', #20745, #37431, #9195 ) ;
#43664=FACE_OUTER_BOUND ( 'NONE', #2046, .T. ) ;
#43665=DIRECTION ( 'NONE',  ( 0.000000000000000000, 0.000000000000000000, -1.000000000000000000 ) ) ;
#43675=AXIS2_PLACEMENT_3D ( 'NONE', #23543, #16339, #46584 ) ;
#43760=ADVANCED_FACE ( 'NONE', ( #13884 ), #9298, .F. ) ;
#43768=EDGE_CURVE ( 'NONE', #35926, #609, #28026, .T. ) ;
#43857=CARTESIAN_POINT ( 'NONE',  ( -15.00000000000000000, 0.000000000000000000, 0.000000000000000000 ) ) ;
#43897=CIRCLE ( 'NONE', #7886, 0.4999999999999992228 ) ;
#43911=CARTESIAN_POINT ( 'NONE',  ( 6.123233995736766282E-16, 28.48684210526315752, 5.000000000000000000 ) ) ;
#44102=DIRECTION ( 'NONE',  ( 0.000000000000000000, 0.000000000000000000, 1.000000000000000000 ) ) ;
#44131=DIRECTION ( 'NONE',  ( 0.000000000000000000, 0.000000000000000000, -1.000000000000000000 ) ) ;
#44132=VECTOR ( 'NONE', #42064, 1000.000000000000000 ) ;
#44144=DIRECTION ( 'NONE',  ( 0.000000000000000000, 0.2223603367690619725, -0.9749645535258958384 ) ) ;
#44186=EDGE_CURVE ( 'NONE', #5556, #5426, #11265, .T. ) ;
#44206=VECTOR ( 'NONE', #19091, 1000.000000000000000 ) ;
#44213=DIRECTION ( 'NONE',  ( -0.000000000000000000, -1.000000000000000000, -0.000000000000000000 ) ) ;
#44338=ORIENTED_EDGE ( 'NONE', *, *, #23050, .F. ) ;
#44352=CYLINDRICAL_SURFACE ( 'NONE', #41202, 0.5000000000000004441 ) ;
#44355=EDGE_CURVE ( 'NONE', #18141, #42504, #3464, .T. ) ;
#44447=AXIS2_PLACEMENT_3D ( 'NONE', #33634, #48220, #45391 ) ;
#44448=EDGE_CURVE ( 'NONE', #23110, #23498, #48543, .T. ) ;
#44459=ORIENTED_EDGE ( 'NONE', *, *, #7273, .F. ) ;
#44473=DIRECTION ( 'NONE',  ( -6.765175596986472868E-16, 0.9749645535258953943, -0.2223603367690637489 ) ) ;
#44491=VERTEX_POINT ( 'NONE', #18307 ) ;
#44533=ORIENTED_EDGE ( 'NONE', *, *, #37829, .F. ) ;
#44579=CARTESIAN_POINT ( 'NONE',  ( 15.00000000000000000, 8.986842105263161073, -18.46084505325461578 ) ) ;
#44644=( GEOMETRIC_REPRESENTATION_CONTEXT ( 3 ) GLOBAL_UNCERTAINTY_ASSIGNED_CONTEXT ( ( #8706 ) ) GLOBAL_UNIT_ASSIGNED_CONTEXT ( ( #5214, #47269, #50411 ) ) REPRESENTATION_CONTEXT ( 'NONE', 'WORKASPACE' ) );
#44778=DIRECTION ( 'NONE',  ( 0.000000000000000000, 1.000000000000000000, 6.938893903907222067E-15 ) ) ;
#44802=EDGE_LOOP ( 'NONE', ( #35368, #27573, #9111, #48219 ) ) ;
#44835=ORIENTED_EDGE ( 'NONE', *, *, #9100, .T. ) ;
#44946=CARTESIAN_POINT ( 'NONE',  ( 15.00000000000000000, -46.51315789473684248, -5.916985404131818171 ) ) ;
#44996=VECTOR ( 'NONE', #46706, 1000.000000000000000 ) ;
#45007=EDGE_CURVE ( 'NONE', #609, #27759, #45, .T. ) ;
#45030=VECTOR ( 'NONE', #8582, 1000.000000000000000 ) ;
#45082=ADVANCED_FACE ( 'NONE', ( #15944 ), #39806, .F. ) ;
#45104=DIRECTION ( 'NONE',  ( 0.000000000000000000, 0.2223603367690619725, -0.9749645535258958384 ) ) ;
#45200=VECTOR ( 'NONE', #45953, 1000.000000000000000 ) ;
#45207=ADVANCED_FACE ( 'NONE', ( #48197 ), #50153, .F. ) ;
#45220=ORIENTED_EDGE ( 'NONE', *, *, #8880, .T. ) ;
#45243=ADVANCED_FACE ( 'NONE', ( #46624 ), #31033, .F. ) ;
#45271=DIRECTION ( 'NONE',  ( -0.000000000000000000, 1.000000000000000000, 0.000000000000000000 ) ) ;
#45281=CIRCLE ( 'NONE', #284, 0.5000000000000004441 ) ;
#45347=CARTESIAN_POINT ( 'NONE',  ( 14.49999999999999822, 12.98684210526315930, -19.37312575500899570 ) ) ;
#45356=ORIENTED_EDGE ( 'NONE', *, *, #13886, .F. ) ;
#45383=AXIS2_PLACEMENT_3D ( 'NONE', #45893, #14378, #10775 ) ;
#45391=DIRECTION ( 'NONE',  ( 1.000000000000000000, 0.000000000000000000, 0.000000000000000000 ) ) ;
#45458=( BOUNDED_CURVE ( )  B_SPLINE_CURVE ( 3, ( #32508, #4282, #47837, #28134 ),
 .UNSPECIFIED., .F., .F. ) 
 B_SPLINE_CURVE_WITH_KNOTS ( ( 4, 4 ),
 ( 4.712388980384684345, 6.058950556070484161 ),
 .UNSPECIFIED. ) 
 CURVE ( )  GEOMETRIC_REPRESENTATION_ITEM ( )  RATIONAL_B_SPLINE_CURVE ( ( 1.000000000000000000, 0.8545200852688803472, 0.8545200852688803472, 1.000000000000000000 ) ) 
 REPRESENTATION_ITEM ( '' )  );
#45486=AXIS2_PLACEMENT_3D ( 'NONE', #31923, #7813, #35026 ) ;
#45587=CARTESIAN_POINT ( 'NONE',  ( 14.49999999999999822, 12.98684210526315930, -19.37312575500900280 ) ) ;
#45626=ORIENTED_EDGE ( 'NONE', *, *, #31534, .T. ) ;
#45634=CARTESIAN_POINT ( 'NONE',  ( 14.49999999999999822, -46.12433806312137108, -6.404467680894764925 ) ) ;
#45658=CARTESIAN_POINT ( 'NONE',  ( -14.49999999999999822, -46.12433806312137108, 6.404467680894761372 ) ) ;
#45682=ORIENTED_EDGE ( 'NONE', *, *, #1240, .T. ) ;
#45784=ADVANCED_FACE ( 'NONE', ( #35093 ), #31743, .T. ) ;
#45785=ORIENTED_EDGE ( 'NONE', *, *, #40037, .T. ) ;
#45839=ORIENTED_EDGE ( 'NONE', *, *, #13997, .T. ) ;
#45893=CARTESIAN_POINT ( 'NONE',  ( 15.00000000000000000, 13.48684210526315930, 20.00000000000000000 ) ) ;
#45953=DIRECTION ( 'NONE',  ( -1.000000000000000000, 0.000000000000000000, 0.000000000000000000 ) ) ;
#46117=VERTEX_POINT ( 'NONE', #50349 ) ;
#46172=EDGE_LOOP ( 'NONE', ( #18471, #21785, #1288, #35239 ) ) ;
#46180=AXIS2_PLACEMENT_3D ( 'NONE', #41196, #1709, #44778 ) ;
#46236=DIRECTION ( 'NONE',  ( 0.000000000000000000, -0.2223603367690619725, 0.9749645535258958384 ) ) ;
#46340=ORIENTED_EDGE ( 'NONE', *, *, #34364, .T. ) ;
#46350=AXIS2_PLACEMENT_3D ( 'NONE', #38902, #27337, #3728 ) ;
#46393=ORIENTED_EDGE ( 'NONE', *, *, #7114, .T. ) ;
#46478=ADVANCED_FACE ( 'NONE', ( #31554 ), #39753, .T. ) ;
#46481=ADVANCED_FACE ( 'NONE', ( #23842 ), #12044, .T. ) ;
#46501=DIRECTION ( 'NONE',  ( 0.000000000000000000, -1.000000000000000000, 0.000000000000000000 ) ) ;
#46516=EDGE_CURVE ( 'NONE', #16307, #32346, #8514, .T. ) ;
#46532=EDGE_CURVE ( 'NONE', #1662, #40121, #36398, .T. ) ;
#46555=ORIENTED_EDGE ( 'NONE', *, *, #47830, .F. ) ;
#46568=CARTESIAN_POINT ( 'NONE',  ( -10.50000000000003730, 13.48684210526314331, -19.99999999999999645 ) ) ;
#46577=CARTESIAN_POINT ( 'NONE',  ( 9.999999999999996447, -34.54492135858216528, 5.000000000000000000 ) ) ;
#46584=DIRECTION ( 'NONE',  ( 1.000000000000000000, 0.000000000000000000, 0.000000000000000000 ) ) ;
#46593=VECTOR ( 'NONE', #28262, 1000.000000000000000 ) ;
#46603=ORIENTED_EDGE ( 'NONE', *, *, #38493, .T. ) ;
#46606=AXIS2_PLACEMENT_3D ( 'NONE', #49682, #8352, #26886 ) ;
#46624=FACE_OUTER_BOUND ( 'NONE', #13943, .T. ) ;
#46706=DIRECTION ( 'NONE',  ( 0.000000000000000000, 0.9749645535258953943, -0.2223603367690637489 ) ) ;
#46726=LINE ( 'NONE', #7526, #24708 ) ;
#46739=ORIENTED_EDGE ( 'NONE', *, *, #7664, .F. ) ;
#46782=VERTEX_POINT ( 'NONE', #48566 ) ;
#46817=ORIENTED_EDGE ( 'NONE', *, *, #7062, .F. ) ;
#46850=CARTESIAN_POINT ( 'NONE',  ( -15.00000000000000000, 12.98684210526315930, 19.37312575500900280 ) ) ;
#46879=VECTOR ( 'NONE', #35204, 1000.000000000000000 ) ;
#46898=CARTESIAN_POINT ( 'NONE',  ( 14.49999999999999822, -46.01315789473684248, -5.916985404131817283 ) ) ;
#46957=ORIENTED_EDGE ( 'NONE', *, *, #33362, .T. ) ;
#46989=ORIENTED_EDGE ( 'NONE', *, *, #39942, .F. ) ;
#47000=CARTESIAN_POINT ( 'NONE',  ( 14.49999999999999822, 13.48684210526315930, 19.37312575500900280 ) ) ;
#47039=ORIENTED_EDGE ( 'NONE', *, *, #25079, .T. ) ;
#47130=DIRECTION ( 'NONE',  ( 1.734723475976805319E-15, 0.000000000000000000, 1.000000000000000000 ) ) ;
#47195=EDGE_CURVE ( 'NONE', #3066, #19764, #12865, .T. ) ;
#47257=PRODUCT_DEFINITION_CONTEXT ( 'detailed design', #20728, 'design' ) ;
#47269=( NAMED_UNIT ( * ) PLANE_ANGLE_UNIT ( ) SI_UNIT ( $, .RADIAN. ) );
#47280=FACE_OUTER_BOUND ( 'NONE', #19567, .T. ) ;
#47291=ADVANCED_FACE ( 'NONE', ( #38755, #18212 ), #11293, .F. ) ;
#47323=ORIENTED_EDGE ( 'NONE', *, *, #24926, .T. ) ;
#47339=DIRECTION ( 'NONE',  ( 0.000000000000000000, 1.000000000000000000, 0.000000000000000000 ) ) ;
#47376=CARTESIAN_POINT ( 'NONE',  ( -10.49999999999999467, -46.51315789473684248, -5.916985404131818171 ) ) ;
#47407=CARTESIAN_POINT ( 'NONE',  ( 14.49999999999999822, -46.01315789473684248, 0.000000000000000000 ) ) ;
#47436=CIRCLE ( 'NONE', #37643, 0.5000000000000004441 ) ;
#47440=EDGE_CURVE ( 'NONE', #12400, #16599, #9268, .T. ) ;
#47465=DIRECTION ( 'NONE',  ( 1.542934785277601468E-15, -0.9749645535258959494, -0.2223603367690620558 ) ) ;
#47474=CARTESIAN_POINT ( 'NONE',  ( 15.00000000000000000, 13.48684210526315930, -19.37312575500899570 ) ) ;
#47478=CIRCLE ( 'NONE', #13079, 0.5000000000000004441 ) ;
#47541=FACE_OUTER_BOUND ( 'NONE', #27622, .T. ) ;
#47620=CARTESIAN_POINT ( 'NONE',  ( -14.49999999999999822, 12.98684210526315930, -19.37312575500900280 ) ) ;
#47687=ORIENTED_EDGE ( 'NONE', *, *, #14539, .T. ) ;
#47707=LINE ( 'NONE', #12592, #46593 ) ;
#47730=ORIENTED_EDGE ( 'NONE', *, *, #28054, .T. ) ;
#47742=EDGE_CURVE ( 'NONE', #10525, #28510, #20758, .T. ) ;
#47770=LINE ( 'NONE', #36797, #28837 ) ;
#47797=CIRCLE ( 'NONE', #42107, 5.000000000000000888 ) ;
#47801=ORIENTED_EDGE ( 'NONE', *, *, #19007, .F. ) ;
#47807=VERTEX_POINT ( 'NONE', #50430 ) ;
#47811=ADVANCED_FACE ( 'NONE', ( #7900 ), #34851, .T. ) ;
#47830=EDGE_CURVE ( 'NONE', #1161, #37697, #32241, .T. ) ;
#47837=CARTESIAN_POINT ( 'NONE',  ( 10.06660411345801620, 8.486842105263159297, 18.70408263333243326 ) ) ;
#47929=ORIENTED_EDGE ( 'NONE', *, *, #16369, .F. ) ;
#47969=CARTESIAN_POINT ( 'NONE',  ( 9.999999999999998224, 8.486842105263161073, 18.34680996553531784 ) ) ;
#48170=CARTESIAN_POINT ( 'NONE',  ( 0.000000000000000000, 13.98684210526316107, 0.000000000000000000 ) ) ;
#48197=FACE_OUTER_BOUND ( 'NONE', #28849, .T. ) ;
#48219=ORIENTED_EDGE ( 'NONE', *, *, #23784, .F. ) ;
#48220=DIRECTION ( 'NONE',  ( 0.000000000000000000, -0.000000000000000000, 1.000000000000000000 ) ) ;
#48273=DIRECTION ( 'NONE',  ( 1.000000000000000000, -0.000000000000000000, -0.000000000000000000 ) ) ;
#48277=AXIS2_PLACEMENT_3D ( 'NONE', #6799, #26307, #30149 ) ;
#48309=DIRECTION ( 'NONE',  ( 0.000000000000000000, 1.000000000000000000, -0.000000000000000000 ) ) ;
#48425=VECTOR ( 'NONE', #44213, 1000.000000000000000 ) ;
#48451=PRODUCT_DEFINITION ( 'UNKNOWN', '', #6196, #47257 ) ;
#48467=ORIENTED_EDGE ( 'NONE', *, *, #17860, .T. ) ;
#48481=DIRECTION ( 'NONE',  ( 0.000000000000000000, -0.2223603367690619725, -0.9749645535258958384 ) ) ;
#48506=ORIENTED_EDGE ( 'NONE', *, *, #8504, .T. ) ;
#48510=CIRCLE ( 'NONE', #21481, 0.5000000000000004441 ) ;
#48543=( BOUNDED_CURVE ( )  B_SPLINE_CURVE ( 3, ( #29621, #6285, #24837, #13958 ),
 .UNSPECIFIED., .F., .F. ) 
 B_SPLINE_CURVE_WITH_KNOTS ( ( 4, 4 ),
 ( 0.2242347511090958534, 1.570796326794895670 ),
 .UNSPECIFIED. ) 
 CURVE ( )  GEOMETRIC_REPRESENTATION_ITEM ( )  RATIONAL_B_SPLINE_CURVE ( ( 1.000000000000000000, 0.8545200852688803472, 0.8545200852688803472, 1.000000000000000000 ) ) 
 REPRESENTATION_ITEM ( '' )  );
#48559=APPLICATION_CONTEXT ( 'automotive_design' ) ;
#48566=CARTESIAN_POINT ( 'NONE',  ( -15.00000000000000000, -46.01315789473684248, -5.916985404131814619 ) ) ;
#48599=CARTESIAN_POINT ( 'NONE',  ( 9.999999999999998224, 8.486842105263161073, 18.34680996553531784 ) ) ;
#48635=CARTESIAN_POINT ( 'NONE',  ( 14.49999999999999822, 12.98684210526315930, -19.37312575500900280 ) ) ;
#48649=ORIENTED_EDGE ( 'NONE', *, *, #42744, .T. ) ;
#48676=FACE_OUTER_BOUND ( 'NONE', #38163, .T. ) ;
#48692=EDGE_LOOP ( 'NONE', ( #2662, #41545, #47323, #49847 ) ) ;
#48702=CARTESIAN_POINT ( 'NONE',  ( -14.49999999999999822, 12.98684210526315930, 20.00000000000000000 ) ) ;
#48710=FACE_OUTER_BOUND ( 'NONE', #7325, .T. ) ;
#48792=ORIENTED_EDGE ( 'NONE', *, *, #32682, .T. ) ;
#48815=CARTESIAN_POINT ( 'NONE',  ( 15.00000000000000000, -3.557843729863133575, 15.59977635401528673 ) ) ;
#48998=ORIENTED_EDGE ( 'NONE', *, *, #38757, .F. ) ;
#49049=CARTESIAN_POINT ( 'NONE',  ( 14.49999999999999822, 13.48684210526315930, -19.37312575500899570 ) ) ;
#49075=DIRECTION ( 'NONE',  ( 0.000000000000000000, 0.9749645535258950613, -0.2223603367690656918 ) ) ;
#49112=AXIS2_PLACEMENT_3D ( 'NONE', #23205, #39631, #31176 ) ;
#49122=DIRECTION ( 'NONE',  ( 0.000000000000000000, 0.000000000000000000, 1.000000000000000000 ) ) ;
#49152=ORIENTED_EDGE ( 'NONE', *, *, #7056, .T. ) ;
#49170=ORIENTED_EDGE ( 'NONE', *, *, #10770, .T. ) ;
#49171=CARTESIAN_POINT ( 'NONE',  ( -10.00419011302953187, 8.486842105263161073, 18.42339408367722697 ) ) ;
#49274=DIRECTION ( 'NONE',  ( -1.000000000000000000, 0.000000000000000000, 0.000000000000000000 ) ) ;
#49289=DIRECTION ( 'NONE',  ( -0.000000000000000000, -0.000000000000000000, -1.000000000000000000 ) ) ;
#49300=CYLINDRICAL_SURFACE ( 'NONE', #4626, 0.5000000000000004441 ) ;
#49321=DIRECTION ( 'NONE',  ( 0.000000000000000000, 0.000000000000000000, 1.000000000000000000 ) ) ;
#49360=EDGE_LOOP ( 'NONE', ( #1555, #39808, #43041, #49788 ) ) ;
#49418=CARTESIAN_POINT ( 'NONE',  ( 0.000000000000000000, 23.48684210526316107, 0.000000000000000000 ) ) ;
#49488=VERTEX_POINT ( 'NONE', #22404 ) ;
#49499=CARTESIAN_POINT ( 'NONE',  ( 15.00000000000000000, 12.98684210526315930, 19.37312575500900280 ) ) ;
#49533=CIRCLE ( 'NONE', #30732, 0.4999999999999997224 ) ;
#49596=DIRECTION ( 'NONE',  ( 0.000000000000000000, 0.000000000000000000, 1.000000000000000000 ) ) ;
#49630=CARTESIAN_POINT ( 'NONE',  ( -15.00000000000000000, 12.98684210526315930, -19.37312575500900280 ) ) ;
#49682=CARTESIAN_POINT ( 'NONE',  ( 10.50000000000000178, -46.01315789473684248, 5.916985404131810178 ) ) ;
#49729=DIRECTION ( 'NONE',  ( 0.000000000000000000, -0.2223603367690619725, -0.9749645535258958384 ) ) ;
#49788=ORIENTED_EDGE ( 'NONE', *, *, #28725, .F. ) ;
#49847=ORIENTED_EDGE ( 'NONE', *, *, #24579, .T. ) ;
#49886=EDGE_CURVE ( 'NONE', #9479, #34755, #7780, .T. ) ;
#49924=DIRECTION ( 'NONE',  ( -1.000000000000000000, 0.000000000000000000, -0.000000000000000000 ) ) ;
#50036=CARTESIAN_POINT ( 'NONE',  ( 0.000000000000000000, 28.48684210526315752, -5.000000000000000000 ) ) ;
#50058=CARTESIAN_POINT ( 'NONE',  ( 15.00000000000000000, 12.98684210526315930, -19.37312575500900280 ) ) ;
#50075=ADVANCED_FACE ( 'NONE', ( #21711 ), #25571, .T. ) ;
#50079=( BOUNDED_CURVE ( )  B_SPLINE_CURVE ( 3, ( #2264, #49171, #6366, #26378 ),
 .UNSPECIFIED., .F., .F. ) 
 B_SPLINE_CURVE_WITH_KNOTS ( ( 4, 4 ),
 ( 1.346561575685801593, 1.570796326794899667 ),
 .UNSPECIFIED. ) 
 CURVE ( )  GEOMETRIC_REPRESENTATION_ITEM ( )  RATIONAL_B_SPLINE_CURVE ( ( 1.000000000000000000, 0.9958142854328206894, 0.9958142854328206894, 1.000000000000000000 ) ) 
 REPRESENTATION_ITEM ( '' )  );
#50096=CARTESIAN_POINT ( 'NONE',  ( 0.000000000000000000, 28.48684210526315752, 0.000000000000000000 ) ) ;
#50145=CARTESIAN_POINT ( 'NONE',  ( -10.49999999999999467, -46.12433806312137108, 6.404467680894761372 ) ) ;
#50153=TOROIDAL_SURFACE ( 'NONE', #42838, 4.250000000000000000, 0.5000000000000000000 ) ;
#50199=CIRCLE ( 'NONE', #42050, 0.5000000000000004441 ) ;
#50233=AXIS2_PLACEMENT_3D ( 'NONE', #25920, #13832, #10004 ) ;
#50333=EDGE_CURVE ( 'NONE', #5824, #42182, #49533, .T. ) ;
#50349=CARTESIAN_POINT ( 'NONE',  ( 0.000000000000000000, 28.48684210526315752, -5.000000000000000000 ) ) ;
#50383=CIRCLE ( 'NONE', #6998, 0.4999999999999992228 ) ;
#50411=( NAMED_UNIT ( * ) SI_UNIT ( $, .STERADIAN. ) SOLID_ANGLE_UNIT ( ) );
#50427=CARTESIAN_POINT ( 'NONE',  ( 14.49999999999999822, 13.48684210526315930, -20.00000000000000000 ) ) ;
#50430=CARTESIAN_POINT ( 'NONE',  ( 5.204748896376250699E-16, 13.48684210526315930, 4.250000000000000000 ) ) ;
#50460=CIRCLE ( 'NONE', #28395, 0.5000000000000004441 ) ;
#50498=FACE_OUTER_BOUND ( 'NONE', #32897, .T. ) ;
#50519=ORIENTED_EDGE ( 'NONE', *, *, #9570, .F. ) ;
#50614=CARTESIAN_POINT ( 'NONE',  ( 0.000000000000000000, 23.48684210526316107, 0.000000000000000000 ) ) ;
#50670=CYLINDRICAL_SURFACE ( 'NONE', #4828, 0.4999999999999992228 ) ;
#50677=DIRECTION ( 'NONE',  ( -0.000000000000000000, -0.9749645535258953943, 0.2223603367690637489 ) ) ;
#50720=CARTESIAN_POINT ( 'NONE',  ( -14.49999999999999822, -46.01315789473684248, -5.916985404131817283 ) ) ;
#50769=COLOUR_RGB('Black',0.12,0.14,0.17);
#50770=FILL_AREA_STYLE_COLOUR('',#50769);
#50771=FILL_AREA_STYLE('',(#50770));
#50772=SURFACE_STYLE_FILL_AREA(#50771);
#50773=SURFACE_SIDE_STYLE('',(#50772));
#50774=SURFACE_STYLE_USAGE(.BOTH.,#50773);
#50775=PRESENTATION_STYLE_ASSIGNMENT((#50774));
ENDSEC;
END-ISO-10303-21;
